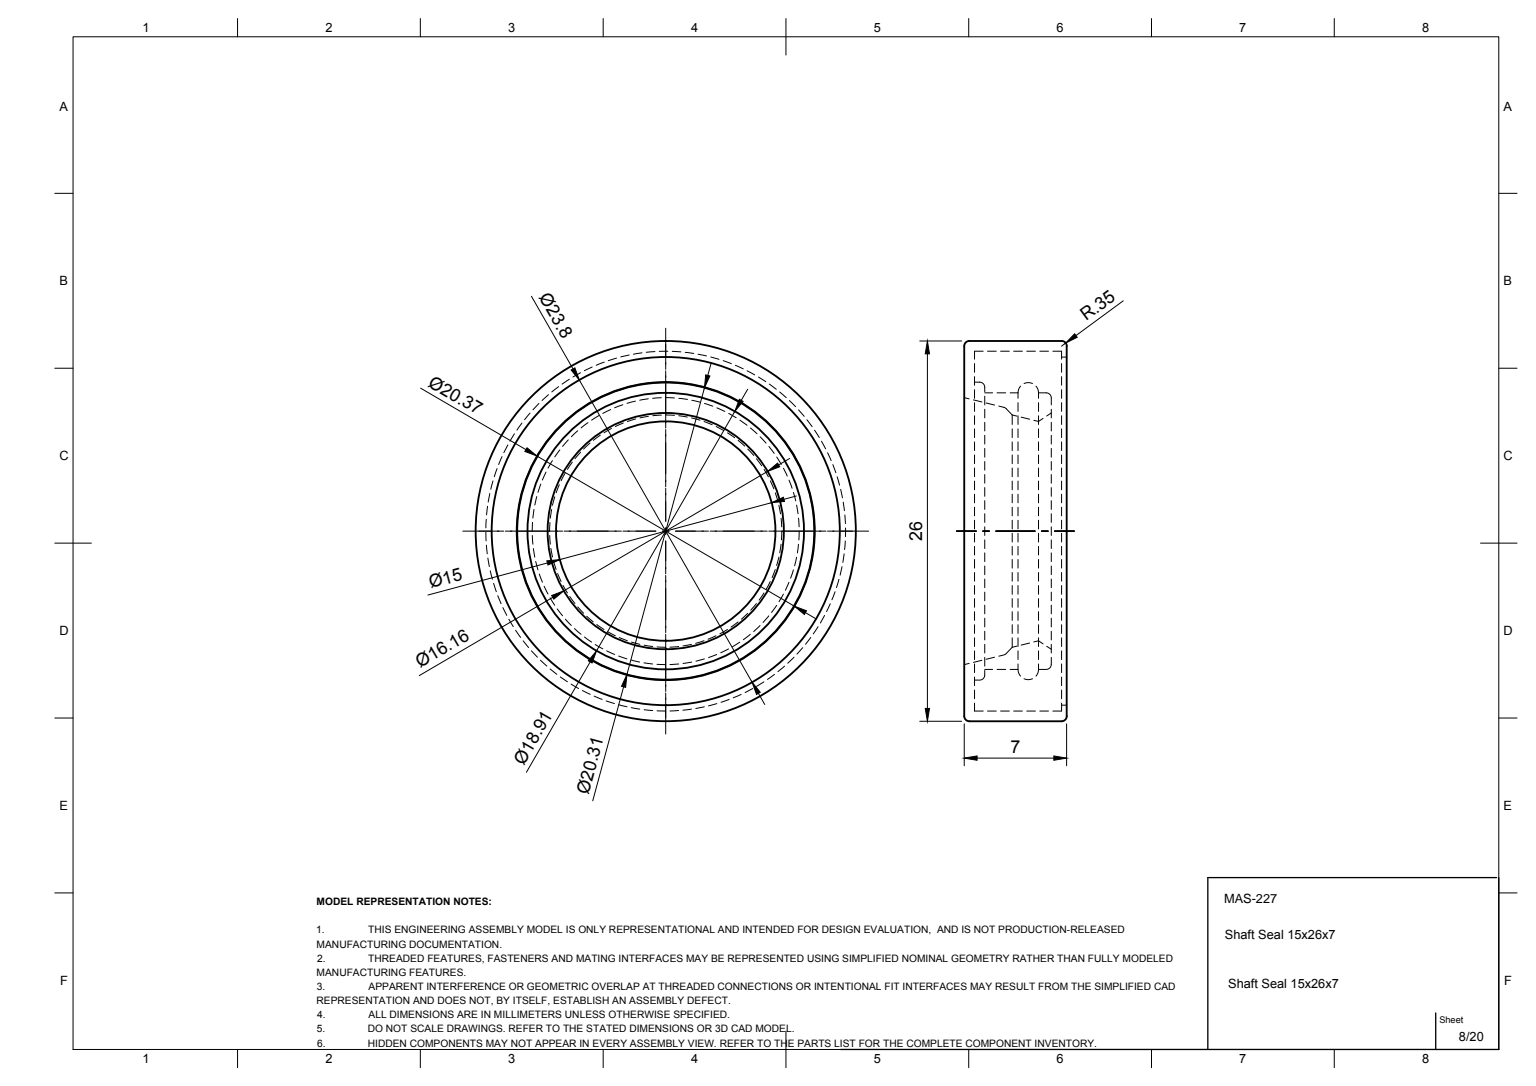
ISO-10303-21;
HEADER;
FILE_DESCRIPTION (('STEP AP214'),
    '1' );
FILE_NAME ( 'Shaft Seal 15x26x7.step', '2026-10-06T08:24:41', ( '' ), ( '' ), 'STEP AP214', 'Unspecified', '' );
FILE_SCHEMA (( 'AUTOMOTIVE_DESIGN' ));
ENDSEC;
DATA;
#41=DIRECTION ( 'NONE',  ( 0.000000000000000000, 0.000000000000000000, -1.000000000000000000 ) ) ;
#65=CARTESIAN_POINT ( 'NONE',  ( 0.000000000000000000, 0.000000000000000000, -0.2618110236220472231 ) ) ;
#81=EDGE_CURVE ( 'NONE', #10766, #14002, #19559, .T. ) ;
#117=DIRECTION ( 'NONE',  ( -1.000000000000000000, 0.000000000000000000, 0.000000000000000000 ) ) ;
#194=CARTESIAN_POINT ( 'NONE',  ( 0.000000000000000000, 0.000000000000000000, -0.2204724409448818867 ) ) ;
#212=AXIS2_PLACEMENT_3D ( 'NONE', #21327, #27824, #8463 ) ;
#213=ORIENTED_EDGE ( 'NONE', *, *, #16639, .F. ) ;
#238=SURFACE_STYLE_USAGE ( .BOTH. , #19827 ) ;
#254=CARTESIAN_POINT ( 'NONE',  ( 0.3722026523000413478, 4.558167867734008572E-17, -0.07578740157480315376 ) ) ;
#265=CIRCLE ( 'NONE', #4300, 0.01377952755905510404 ) ;
#273=AXIS2_PLACEMENT_3D ( 'NONE', #1316, #18082, #27170 ) ;
#296=EDGE_CURVE ( 'NONE', #10766, #14592, #15963, .T. ) ;
#303=DIRECTION ( 'NONE',  ( 0.000000000000000000, 0.000000000000000000, -1.000000000000000000 ) ) ;
#331=CARTESIAN_POINT ( 'NONE',  ( 0.000000000000000000, 0.000000000000000000, -0.2342519685039370358 ) ) ;
#348=EDGE_CURVE ( 'NONE', #27369, #9997, #27259, .T. ) ;
#359=DIRECTION ( 'NONE',  ( -1.000000000000000000, -1.224646799147356165E-16, 0.000000000000000000 ) ) ;
#376=CYLINDRICAL_SURFACE ( 'NONE', #17012, 0.4842519685039370358 ) ;
#434=DIRECTION ( 'NONE',  ( -1.000000000000000000, 0.000000000000000000, 0.000000000000000000 ) ) ;
#439=EDGE_LOOP ( 'NONE', ( #13382, #10561, #4608, #2891 ) ) ;
#443=CARTESIAN_POINT ( 'NONE',  ( 0.3066721922917531873, -3.755651186775971117E-17, -0.05856299212598425896 ) ) ;
#487=PRESENTATION_STYLE_ASSIGNMENT (( #238 ) ) ;
#499=DIRECTION ( 'NONE',  ( 0.000000000000000000, 0.000000000000000000, -1.000000000000000000 ) ) ;
#520=EDGE_LOOP ( 'NONE', ( #11696, #24909 ) ) ;
#533=ORIENTED_EDGE ( 'NONE', *, *, #26084, .F. ) ;
#592=ORIENTED_EDGE ( 'NONE', *, *, #21913, .F. ) ;
#630=TOROIDAL_SURFACE ( 'NONE', #15950, 0.3198827364362346048, 0.01377952755905511792 ) ;
#645=AXIS2_PLACEMENT_3D ( 'NONE', #18436, #14238, #22419 ) ;
#669=PRODUCT_DEFINITION ( 'UNKNOWN', '', #23773, #14490 ) ;
#675=EDGE_CURVE ( 'NONE', #10287, #12118, #11029, .T. ) ;
#684=AXIS2_PLACEMENT_3D ( 'NONE', #21009, #24675, #18877 ) ;
#749=DIRECTION ( 'NONE',  ( 0.000000000000000000, 0.000000000000000000, -1.000000000000000000 ) ) ;
#751=EDGE_CURVE ( 'NONE', #9997, #27369, #23688, .T. ) ;
#795=EDGE_LOOP ( 'NONE', ( #9740, #5198 ) ) ;
#821=DIRECTION ( 'NONE',  ( 0.000000000000000000, 0.000000000000000000, -1.000000000000000000 ) ) ;
#831=TOROIDAL_SURFACE ( 'NONE', #22041, 0.3584231247409862542, 0.01377952755905511792 ) ;
#855=AXIS2_PLACEMENT_3D ( 'NONE', #18013, #5044, #5477 ) ;
#862=EDGE_CURVE ( 'NONE', #24185, #27369, #15261, .T. ) ;
#879=ORIENTED_EDGE ( 'NONE', *, *, #17592, .T. ) ;
#923=ORIENTED_EDGE ( 'NONE', *, *, #17887, .T. ) ;
#963=LINE ( 'NONE', #9553, #16645 ) ;
#993=AXIS2_PLACEMENT_3D ( 'NONE', #65, #8764, #25589 ) ;
#1001=EDGE_CURVE ( 'NONE', #12118, #10287, #27735, .T. ) ;
#1023=ORIENTED_EDGE ( 'NONE', *, *, #2966, .T. ) ;
#1035=ORIENTED_EDGE ( 'NONE', *, *, #1061, .T. ) ;
#1038=AXIS2_PLACEMENT_3D ( 'NONE', #13010, #9304, #25877 ) ;
#1061=EDGE_CURVE ( 'NONE', #11368, #24827, #15560, .T. ) ;
#1071=EDGE_CURVE ( 'NONE', #14592, #10766, #7407, .T. ) ;
#1096=EDGE_CURVE ( 'NONE', #24517, #18812, #4630, .T. ) ;
#1103=CARTESIAN_POINT ( 'NONE',  ( -0.3066721922917531873, 0.000000000000000000, -0.05856299212598425896 ) ) ;
#1164=FACE_OUTER_BOUND ( 'NONE', #3351, .T. ) ;
#1242=EDGE_LOOP ( 'NONE', ( #16794, #2990 ) ) ;
#1270=FACE_OUTER_BOUND ( 'NONE', #4883, .T. ) ;
#1292=CIRCLE ( 'NONE', #4886, 0.5118110236220472231 ) ;
#1316=CARTESIAN_POINT ( 'NONE',  ( 0.000000000000000000, 0.000000000000000000, -0.05511811023622047168 ) ) ;
#1322=CARTESIAN_POINT ( 'NONE',  ( -0.3451357231661831282, 0.000000000000000000, -0.04133858267716535029 ) ) ;
#1325=VERTEX_POINT ( 'NONE', #15223 ) ;
#1343=EDGE_CURVE ( 'NONE', #22371, #24517, #19627, .T. ) ;
#1436=DIRECTION ( 'NONE',  ( 0.000000000000000000, 0.000000000000000000, -1.000000000000000000 ) ) ;
#1440=DIRECTION ( 'NONE',  ( 0.000000000000000000, 0.000000000000000000, -1.000000000000000000 ) ) ;
#1451=DIRECTION ( 'NONE',  ( -1.000000000000000000, 0.000000000000000000, 0.000000000000000000 ) ) ;
#1459=DIRECTION ( 'NONE',  ( -1.000000000000000000, 0.000000000000000000, 0.000000000000000000 ) ) ;
#1475=EDGE_LOOP ( 'NONE', ( #26767, #10716, #19172, #19322 ) ) ;
#1521=ORIENTED_EDGE ( 'NONE', *, *, #22805, .F. ) ;
#1534=EDGE_LOOP ( 'NONE', ( #26895, #14116, #21082, #6619 ) ) ;
#1556=CIRCLE ( 'NONE', #7876, 0.01377952755905510404 ) ;
#1607=CARTESIAN_POINT ( 'NONE',  ( 0.3294268239828485600, 4.034315055438739563E-17, -0.1625845656552793450 ) ) ;
#1612=ORIENTED_EDGE ( 'NONE', *, *, #7598, .F. ) ;
#1664=ORIENTED_EDGE ( 'NONE', *, *, #21562, .F. ) ;
#1690=DIRECTION ( 'NONE',  ( 0.000000000000000000, 0.000000000000000000, -1.000000000000000000 ) ) ;
#1736=DIRECTION ( 'NONE',  ( 0.000000000000000000, 0.000000000000000000, -1.000000000000000000 ) ) ;
#1759=FACE_OUTER_BOUND ( 'NONE', #17673, .T. ) ;
#1765=DIRECTION ( 'NONE',  ( 0.000000000000000000, 0.000000000000000000, -1.000000000000000000 ) ) ;
#1780=CARTESIAN_POINT ( 'NONE',  ( -0.4842519685039370358, 0.000000000000000000, -0.2480314960629921295 ) ) ;
#1842=LINE ( 'NONE', #25717, #22886 ) ;
#1850=EDGE_CURVE ( 'NONE', #14002, #24185, #9702, .T. ) ;
#1887=ORIENTED_EDGE ( 'NONE', *, *, #14871, .F. ) ;
#1940=EDGE_LOOP ( 'NONE', ( #3671, #24447, #23194, #8528 ) ) ;
#1952=VERTEX_POINT ( 'NONE', #2654 ) ;
#1999=VECTOR ( 'NONE', #24433, 39.37007874015748854 ) ;
#2097=ORIENTED_EDGE ( 'NONE', *, *, #16708, .F. ) ;
#2112=CARTESIAN_POINT ( 'NONE',  ( -0.3872945158171015589, 0.000000000000000000, -0.2204724409448818867 ) ) ;
#2132=CARTESIAN_POINT ( 'NONE',  ( -0.3722026523000413478, 0.000000000000000000, -0.1033464566929133965 ) ) ;
#2163=CARTESIAN_POINT ( 'NONE',  ( -0.5118110236220472231, 0.000000000000000000, -0.2618110236220472231 ) ) ;
#2169=ORIENTED_EDGE ( 'NONE', *, *, #348, .F. ) ;
#2180=AXIS2_PLACEMENT_3D ( 'NONE', #21071, #20654, #10050 ) ;
#2191=CARTESIAN_POINT ( 'NONE',  ( 0.000000000000000000, 0.000000000000000000, -0.2618110236220472231 ) ) ;
#2199=AXIS2_PLACEMENT_3D ( 'NONE', #24532, #20307, #18304 ) ;
#2320=FACE_OUTER_BOUND ( 'NONE', #11386, .T. ) ;
#2334=DIRECTION ( 'NONE',  ( -0.000000000000000000, -1.000000000000000000, -0.000000000000000000 ) ) ;
#2335=ORIENTED_EDGE ( 'NONE', *, *, #25585, .F. ) ;
#2415=ADVANCED_FACE ( 'NONE', ( #26187 ), #7944, .T. ) ;
#2529=ORIENTED_EDGE ( 'NONE', *, *, #26084, .T. ) ;
#2537=FACE_OUTER_BOUND ( 'NONE', #20320, .T. ) ;
#2594=DIRECTION ( 'NONE',  ( 0.000000000000000000, 0.000000000000000000, -1.000000000000000000 ) ) ;
#2606=ORIENTED_EDGE ( 'NONE', *, *, #23570, .F. ) ;
#2654=CARTESIAN_POINT ( 'NONE',  ( 0.4842519685039370358, 5.930376232091513698E-17, -0.2480314960629921295 ) ) ;
#2670=CIRCLE ( 'NONE', #22528, 0.4980314960629921295 ) ;
#2764=AXIS2_PLACEMENT_3D ( 'NONE', #194, #11024, #26267 ) ;
#2766=CARTESIAN_POINT ( 'NONE',  ( 0.000000000000000000, 0.000000000000000000, -0.01377952755905511792 ) ) ;
#2803=DIRECTION ( 'NONE',  ( -1.000000000000000000, 0.000000000000000000, 0.000000000000000000 ) ) ;
#2811=AXIS2_PLACEMENT_3D ( 'NONE', #14470, #19390, #16714 ) ;
#2837=AXIS2_PLACEMENT_3D ( 'NONE', #4234, #8058, #16514 ) ;
#2841=CARTESIAN_POINT ( 'NONE',  ( -0.3584231247409862542, 0.000000000000000000, -0.05511811023622047168 ) ) ;
#2868=DIRECTION ( 'NONE',  ( 0.000000000000000000, 0.000000000000000000, -1.000000000000000000 ) ) ;
#2891=ORIENTED_EDGE ( 'NONE', *, *, #7871, .F. ) ;
#2901=AXIS2_PLACEMENT_3D ( 'NONE', #27696, #24860, #14143 ) ;
#2907=DIRECTION ( 'NONE',  ( 0.000000000000000000, 0.000000000000000000, -1.000000000000000000 ) ) ;
#2925=( NAMED_UNIT ( * ) PLANE_ANGLE_UNIT ( ) SI_UNIT ( $, .RADIAN. ) ) ;
#2931=ORIENTED_EDGE ( 'NONE', *, *, #15459, .F. ) ;
#2966=EDGE_CURVE ( 'NONE', #10287, #1952, #26468, .T. ) ;
#2990=ORIENTED_EDGE ( 'NONE', *, *, #13862, .F. ) ;
#3078=DIRECTION ( 'NONE',  ( -1.000000000000000000, 0.000000000000000000, 0.000000000000000000 ) ) ;
#3085=UNCERTAINTY_MEASURE_WITH_UNIT (LENGTH_MEASURE( 1.000000000000000082E-05 ), #4516, 'distance_accuracy_value', 'NONE') ;
#3099=AXIS2_PLACEMENT_3D ( 'NONE', #25907, #6556, #5249 ) ;
#3113=DIRECTION ( 'NONE',  ( -1.000000000000000000, 0.000000000000000000, 0.000000000000000000 ) ) ;
#3117=VERTEX_POINT ( 'NONE', #26939 ) ;
#3156=CARTESIAN_POINT ( 'NONE',  ( 0.3722026523000413478, 4.558167867734008572E-17, -0.1756889763779527769 ) ) ;
#3246=LINE ( 'NONE', #11888, #10154 ) ;
#3260=EDGE_CURVE ( 'NONE', #24896, #24517, #12074, .T. ) ;
#3264=ORIENTED_EDGE ( 'NONE', *, *, #19902, .T. ) ;
#3351=EDGE_LOOP ( 'NONE', ( #1612, #533, #23574, #1035 ) ) ;
#3364=CIRCLE ( 'NONE', #24588, 0.4685039370078740717 ) ;
#3375=DIRECTION ( 'NONE',  ( -1.224646799147353207E-16, 1.000000000000000000, 0.000000000000000000 ) ) ;
#3414=CARTESIAN_POINT ( 'NONE',  ( 0.4010740433761567081, 4.911740434416970370E-17, -0.2480314960629921295 ) ) ;
#3449=PRODUCT ( 'Shaft Seal 15x26x7', 'Shaft Seal 15x26x7', '', ( #15092 ) ) ;
#3500=EDGE_CURVE ( 'NONE', #23791, #1325, #26299, .T. ) ;
#3545=CONICAL_SURFACE ( 'NONE', #3099, 0.3224687058348476576, 0.8056700744428512140 ) ;
#3574=ADVANCED_FACE ( 'NONE', ( #8255 ), #831, .T. ) ;
#3605=LINE ( 'NONE', #16340, #11324 ) ;
#3619=DIRECTION ( 'NONE',  ( 0.000000000000000000, 0.000000000000000000, -1.000000000000000000 ) ) ;
#3632=CARTESIAN_POINT ( 'NONE',  ( 0.000000000000000000, 0.000000000000000000, -0.2480314960629921295 ) ) ;
#3665=DIRECTION ( 'NONE',  ( 0.000000000000000000, 0.000000000000000000, 1.000000000000000000 ) ) ;
#3671=ORIENTED_EDGE ( 'NONE', *, *, #6583, .T. ) ;
#3747=AXIS2_PLACEMENT_3D ( 'NONE', #13845, #13696, #27128 ) ;
#3757=DIRECTION ( 'NONE',  ( 1.000000000000000000, 0.000000000000000000, 0.000000000000000000 ) ) ;
#3774=CARTESIAN_POINT ( 'NONE',  ( 0.000000000000000000, 0.000000000000000000, -0.2342519685039370358 ) ) ;
#3782=VERTEX_POINT ( 'NONE', #27226 ) ;
#3860=ORIENTED_EDGE ( 'NONE', *, *, #12938, .F. ) ;
#3869=AXIS2_PLACEMENT_3D ( 'NONE', #13603, #22220, #24208 ) ;
#3928=DIRECTION ( 'NONE',  ( -1.000000000000000000, 0.000000000000000000, 0.000000000000000000 ) ) ;
#3959=FACE_BOUND ( 'NONE', #21442, .T. ) ;
#3969=ADVANCED_FACE ( 'NONE', ( #25527 ), #18427, .T. ) ;
#3988=AXIS2_PLACEMENT_3D ( 'NONE', #5088, #13709, #17926 ) ;
#4011=VECTOR ( 'NONE', #2594, 39.37007874015748143 ) ;
#4034=ORIENTED_EDGE ( 'NONE', *, *, #13927, .F. ) ;
#4073=EDGE_LOOP ( 'NONE', ( #12359, #15976, #13179, #213 ) ) ;
#4076=ORIENTED_EDGE ( 'NONE', *, *, #6993, .T. ) ;
#4085=DIRECTION ( 'NONE',  ( 0.000000000000000000, 0.000000000000000000, -1.000000000000000000 ) ) ;
#4131=ORIENTED_EDGE ( 'NONE', *, *, #8880, .F. ) ;
#4152=EDGE_CURVE ( 'NONE', #18288, #1952, #14403, .T. ) ;
#4159=EDGE_CURVE ( 'NONE', #12825, #16461, #23873, .T. ) ;
#4174=DIRECTION ( 'NONE',  ( -1.000000000000000000, 0.000000000000000000, 0.000000000000000000 ) ) ;
#4185=EDGE_CURVE ( 'NONE', #24622, #11368, #963, .T. ) ;
#4198=DIRECTION ( 'NONE',  ( 1.000000000000000000, 0.000000000000000000, 0.000000000000000000 ) ) ;
#4205=VERTEX_POINT ( 'NONE', #11407 ) ;
#4234=CARTESIAN_POINT ( 'NONE',  ( 0.000000000000000000, 0.000000000000000000, -0.04133858267716535029 ) ) ;
#4243=ORIENTED_EDGE ( 'NONE', *, *, #3500, .T. ) ;
#4258=EDGE_CURVE ( 'NONE', #24011, #9956, #2670, .T. ) ;
#4300=AXIS2_PLACEMENT_3D ( 'NONE', #16529, #3375, #25007 ) ;
#4306=LENGTH_MEASURE_WITH_UNIT ( LENGTH_MEASURE( 0.02539999999999999897 ), #16546 ) ;
#4362=FACE_BOUND ( 'NONE', #16942, .T. ) ;
#4391=TOROIDAL_SURFACE ( 'NONE', #13855, 0.4980314960629921295, 0.01377952755905511792 ) ;
#4495=ORIENTED_EDGE ( 'NONE', *, *, #4565, .F. ) ;
#4514=ORIENTED_EDGE ( 'NONE', *, *, #12938, .T. ) ;
#4516=( CONVERSION_BASED_UNIT ( 'INCH', #17637 ) LENGTH_UNIT ( ) NAMED_UNIT ( #13045 ) ) ;
#4522=AXIS2_PLACEMENT_3D ( 'NONE', #23164, #4085, #12689 ) ;
#4543=FACE_OUTER_BOUND ( 'NONE', #439, .T. ) ;
#4565=EDGE_CURVE ( 'NONE', #19035, #26909, #23390, .T. ) ;
#4608=ORIENTED_EDGE ( 'NONE', *, *, #25493, .T. ) ;
#4630=LINE ( 'NONE', #11409, #27280 ) ;
#4651=CARTESIAN_POINT ( 'NONE',  ( -0.4980314960629921295, 0.000000000000000000, -0.01377952755905511792 ) ) ;
#4653=AXIS2_PLACEMENT_3D ( 'NONE', #8465, #16949, #17084 ) ;
#4658=DIRECTION ( 'NONE',  ( 0.000000000000000000, 0.000000000000000000, -1.000000000000000000 ) ) ;
#4672=ORIENTED_EDGE ( 'NONE', *, *, #20993, .F. ) ;
#4698=VECTOR ( 'NONE', #25982, 39.37007874015748143 ) ;
#4709=FACE_OUTER_BOUND ( 'NONE', #18885, .T. ) ;
#4717=CARTESIAN_POINT ( 'NONE',  ( 0.4980314960629921295, 6.099126775281109802E-17, -0.2618110236220472231 ) ) ;
#4744=EDGE_CURVE ( 'NONE', #23791, #26519, #25173, .T. ) ;
#4758=DIRECTION ( 'NONE',  ( -1.000000000000000000, 0.000000000000000000, 0.000000000000000000 ) ) ;
#4790=CARTESIAN_POINT ( 'NONE',  ( -0.3872945158171015589, 0.000000000000000000, -0.2342519685039370358 ) ) ;
#4797=DIRECTION ( 'NONE',  ( 0.000000000000000000, 0.000000000000000000, -1.000000000000000000 ) ) ;
#4813=CYLINDRICAL_SURFACE ( 'NONE', #23754, 0.4842519685039370358 ) ;
#4818=PLANE ( 'NONE',  #10795 ) ;
#4883=EDGE_LOOP ( 'NONE', ( #25142, #5686, #879, #22401 ) ) ;
#4886=AXIS2_PLACEMENT_3D ( 'NONE', #20717, #18864, #3757 ) ;
#4900=CIRCLE ( 'NONE', #8520, 0.01377952755905510404 ) ;
#4917=ORIENTED_EDGE ( 'NONE', *, *, #24991, .T. ) ;
#4922=DIRECTION ( 'NONE',  ( 0.000000000000000000, 0.000000000000000000, -1.000000000000000000 ) ) ;
#4938=LINE ( 'NONE', #16481, #5532 ) ;
#4960=ORIENTED_EDGE ( 'NONE', *, *, #17477, .T. ) ;
#4971=DIRECTION ( 'NONE',  ( -1.224646799147353207E-16, 1.000000000000000000, 0.000000000000000000 ) ) ;
#4989=DIRECTION ( 'NONE',  ( -1.000000000000000000, -1.224646799147356165E-16, 0.000000000000000000 ) ) ;
#5022=ORIENTED_EDGE ( 'NONE', *, *, #1850, .F. ) ;
#5038=FACE_OUTER_BOUND ( 'NONE', #20604, .T. ) ;
#5044=DIRECTION ( 'NONE',  ( 0.000000000000000000, 0.000000000000000000, -1.000000000000000000 ) ) ;
#5065=PLANE ( 'NONE',  #10827 ) ;
#5088=CARTESIAN_POINT ( 'NONE',  ( 0.000000000000000000, 0.000000000000000000, -0.2480314960629921295 ) ) ;
#5132=CARTESIAN_POINT ( 'NONE',  ( 0.000000000000000000, 0.000000000000000000, -0.2480314960629921295 ) ) ;
#5142=EDGE_CURVE ( 'NONE', #26728, #9665, #11645, .T. ) ;
#5157=CARTESIAN_POINT ( 'NONE',  ( -0.3180687940157840843, 0.000000000000000000, -0.04133858267716535029 ) ) ;
#5172=DIRECTION ( 'NONE',  ( 0.000000000000000000, 0.000000000000000000, -1.000000000000000000 ) ) ;
#5198=ORIENTED_EDGE ( 'NONE', *, *, #4258, .F. ) ;
#5209=FACE_BOUND ( 'NONE', #24077, .T. ) ;
#5229=CARTESIAN_POINT ( 'NONE',  ( 0.000000000000000000, 0.000000000000000000, 0.000000000000000000 ) ) ;
#5249=DIRECTION ( 'NONE',  ( -1.000000000000000000, 0.000000000000000000, 0.000000000000000000 ) ) ;
#5324=DIRECTION ( 'NONE',  ( 0.000000000000000000, 0.000000000000000000, -1.000000000000000000 ) ) ;
#5362=EDGE_CURVE ( 'NONE', #24896, #5769, #7155, .T. ) ;
#5426=DIRECTION ( 'NONE',  ( 0.000000000000000000, 0.000000000000000000, -1.000000000000000000 ) ) ;
#5435=DIRECTION ( 'NONE',  ( -1.224646799147353207E-16, 1.000000000000000000, 0.000000000000000000 ) ) ;
#5475=ORIENTED_EDGE ( 'NONE', *, *, #19235, .T. ) ;
#5477=DIRECTION ( 'NONE',  ( -1.000000000000000000, 0.000000000000000000, 0.000000000000000000 ) ) ;
#5526=CARTESIAN_POINT ( 'NONE',  ( -0.3294268239828485600, 0.000000000000000000, -0.1625845656552793450 ) ) ;
#5532=VECTOR ( 'NONE', #13554, 39.37007874015748143 ) ;
#5536=CARTESIAN_POINT ( 'NONE',  ( -0.4980314960629921295, 0.000000000000000000, -6.010066929133858501E-17 ) ) ;
#5627=AXIS2_PLACEMENT_3D ( 'NONE', #7311, #11547, #26653 ) ;
#5653=DIRECTION ( 'NONE',  ( 0.000000000000000000, 0.000000000000000000, 1.000000000000000000 ) ) ;
#5668=CYLINDRICAL_SURFACE ( 'NONE', #16513, 0.5118110236220472231 ) ;
#5686=ORIENTED_EDGE ( 'NONE', *, *, #348, .T. ) ;
#5769=VERTEX_POINT ( 'NONE', #2112 ) ;
#5792=DIRECTION ( 'NONE',  ( 0.2384530002628495460, 2.920207035189816837E-17, -0.9711540385879292581 ) ) ;
#5808=ORIENTED_EDGE ( 'NONE', *, *, #17183, .T. ) ;
#5833=CARTESIAN_POINT ( 'NONE',  ( 0.000000000000000000, 0.000000000000000000, -0.1309055118110236116 ) ) ;
#5841=AXIS2_PLACEMENT_3D ( 'NONE', #9381, #11656, #26442 ) ;
#5879=AXIS2_PLACEMENT_3D ( 'NONE', #10428, #19043, #27677 ) ;
#5923=ORIENTED_EDGE ( 'NONE', *, *, #14871, .T. ) ;
#5944=CARTESIAN_POINT ( 'NONE',  ( 0.000000000000000000, 0.000000000000000000, -0.07578740157480315376 ) ) ;
#5950=EDGE_CURVE ( 'NONE', #7273, #4205, #13910, .T. ) ;
#5972=CYLINDRICAL_SURFACE ( 'NONE', #15485, 0.3722026523000413478 ) ;
#5974=CARTESIAN_POINT ( 'NONE',  ( 0.000000000000000000, 0.000000000000000000, -0.07578740157480315376 ) ) ;
#5976=PRODUCT_DEFINITION_SHAPE ( 'NONE', 'NONE',  #669 ) ;
#6046=EDGE_CURVE ( 'NONE', #24011, #26909, #17569, .T. ) ;
#6071=ORIENTED_EDGE ( 'NONE', *, *, #1061, .F. ) ;
#6081=ADVANCED_FACE ( 'NONE', ( #8664 ), #3545, .F. ) ;
#6095=AXIS2_PLACEMENT_3D ( 'NONE', #19887, #2907, #17877 ) ;
#6167=DIRECTION ( 'NONE',  ( 0.000000000000000000, 0.000000000000000000, -1.000000000000000000 ) ) ;
#6215=( GEOMETRIC_REPRESENTATION_CONTEXT ( 3 ) GLOBAL_UNCERTAINTY_ASSIGNED_CONTEXT ( ( #3085 ) ) GLOBAL_UNIT_ASSIGNED_CONTEXT ( ( #4516, #2925, #13530 ) ) REPRESENTATION_CONTEXT ( 'NONE', 'WORKASPACE' ) ) ;
#6217=DIRECTION ( 'NONE',  ( 0.000000000000000000, 0.000000000000000000, -1.000000000000000000 ) ) ;
#6258=ORIENTED_EDGE ( 'NONE', *, *, #6939, .T. ) ;
#6298=ADVANCED_FACE ( 'NONE', ( #24808 ), #21203, .F. ) ;
#6346=CIRCLE ( 'NONE', #22111, 0.3126261861498082495 ) ;
#6408=VECTOR ( 'NONE', #23622, 39.37007874015748143 ) ;
#6511=CARTESIAN_POINT ( 'NONE',  ( 0.000000000000000000, 0.000000000000000000, -0.2755905511811023723 ) ) ;
#6516=DIRECTION ( 'NONE',  ( 0.000000000000000000, 0.000000000000000000, -1.000000000000000000 ) ) ;
#6522=DIRECTION ( 'NONE',  ( -1.000000000000000000, 0.000000000000000000, 0.000000000000000000 ) ) ;
#6549=ADVANCED_FACE ( 'NONE', ( #22241 ), #11271, .F. ) ;
#6556=DIRECTION ( 'NONE',  ( 0.000000000000000000, 0.000000000000000000, -1.000000000000000000 ) ) ;
#6583=EDGE_CURVE ( 'NONE', #25216, #7273, #13982, .T. ) ;
#6619=ORIENTED_EDGE ( 'NONE', *, *, #1343, .T. ) ;
#6642=SHAPE_REPRESENTATION_RELATIONSHIP ( 'NONE' , 'NONE' ,  #25798, #26182 ) ;
#6643=EDGE_LOOP ( 'NONE', ( #22688, #22613, #16731, #9252 ) ) ;
#6647=ORIENTED_EDGE ( 'NONE', *, *, #4744, .F. ) ;
#6698=AXIS2_PLACEMENT_3D ( 'NONE', #2766, #5172, #4758 ) ;
#6772=CARTESIAN_POINT ( 'NONE',  ( 0.000000000000000000, 0.000000000000000000, -0.04133858267716535029 ) ) ;
#6782=CIRCLE ( 'NONE', #5879, 0.4980314960629921295 ) ;
#6810=ORIENTED_EDGE ( 'NONE', *, *, #24229, .T. ) ;
#6817=DIRECTION ( 'NONE',  ( 1.000000000000000000, 0.000000000000000000, 0.000000000000000000 ) ) ;
#6838=ADVANCED_FACE ( 'NONE', ( #5209, #24420 ), #5065, .T. ) ;
#6882=CARTESIAN_POINT ( 'NONE',  ( 0.000000000000000000, 0.000000000000000000, -0.04133858267716535029 ) ) ;
#6908=AXIS2_PLACEMENT_3D ( 'NONE', #331, #22179, #2803 ) ;
#6939=EDGE_CURVE ( 'NONE', #13078, #3782, #9931, .T. ) ;
#6944=CARTESIAN_POINT ( 'NONE',  ( 0.000000000000000000, 0.000000000000000000, -0.05511811023622047168 ) ) ;
#6955=DIRECTION ( 'NONE',  ( 0.000000000000000000, 0.000000000000000000, 1.000000000000000000 ) ) ;
#6961=FACE_BOUND ( 'NONE', #20194, .T. ) ;
#6993=EDGE_CURVE ( 'NONE', #24685, #19453, #6782, .T. ) ;
#7035=DIRECTION ( 'NONE',  ( -0.5518027697606309179, 0.000000000000000000, 0.8339746418713797071 ) ) ;
#7075=CARTESIAN_POINT ( 'NONE',  ( 0.4980314960629921295, 6.183502046875907854E-17, -6.010066929133858501E-17 ) ) ;
#7155=CIRCLE ( 'NONE', #20236, 0.3872945158171015589 ) ;
#7209=CIRCLE ( 'NONE', #9453, 0.4685039370078740717 ) ;
#7216=ORIENTED_EDGE ( 'NONE', *, *, #19235, .F. ) ;
#7240=DIRECTION ( 'NONE',  ( 0.000000000000000000, 0.000000000000000000, -1.000000000000000000 ) ) ;
#7251=DIRECTION ( 'NONE',  ( -1.224646799147353207E-16, 1.000000000000000000, 0.000000000000000000 ) ) ;
#7269=CIRCLE ( 'NONE', #23083, 0.3126261861498082495 ) ;
#7273=VERTEX_POINT ( 'NONE', #10850 ) ;
#7294=ORIENTED_EDGE ( 'NONE', *, *, #18218, .F. ) ;
#7311=CARTESIAN_POINT ( 'NONE',  ( 0.000000000000000000, 0.000000000000000000, -0.01377952755905511792 ) ) ;
#7319=FACE_OUTER_BOUND ( 'NONE', #20969, .T. ) ;
#7335=DIRECTION ( 'NONE',  ( 0.000000000000000000, 0.000000000000000000, -1.000000000000000000 ) ) ;
#7337=LINE ( 'NONE', #20334, #12740 ) ;
#7340=CONICAL_SURFACE ( 'NONE', #1038, 0.3458446900868161200, 0.2407725888118960322 ) ;
#7389=ORIENTED_EDGE ( 'NONE', *, *, #17516, .F. ) ;
#7401=DIRECTION ( 'NONE',  ( 0.000000000000000000, 0.000000000000000000, -1.000000000000000000 ) ) ;
#7407=CIRCLE ( 'NONE', #21421, 0.3584231247409862542 ) ;
#7429=ORIENTED_EDGE ( 'NONE', *, *, #14472, .F. ) ;
#7435=AXIS2_PLACEMENT_3D ( 'NONE', #21554, #26202, #17317 ) ;
#7573=ORIENTED_EDGE ( 'NONE', *, *, #4152, .F. ) ;
#7598=EDGE_CURVE ( 'NONE', #20206, #24827, #3605, .T. ) ;
#7620=ORIENTED_EDGE ( 'NONE', *, *, #296, .F. ) ;
#7772=DIRECTION ( 'NONE',  ( 0.000000000000000000, 0.000000000000000000, 1.000000000000000000 ) ) ;
#7828=CONICAL_SURFACE ( 'NONE', #17300, 0.3039508883504944969, 0.2407725888118948110 ) ;
#7871=EDGE_CURVE ( 'NONE', #18812, #10946, #13575, .T. ) ;
#7876=AXIS2_PLACEMENT_3D ( 'NONE', #8330, #25560, #6217 ) ;
#7895=ORIENTED_EDGE ( 'NONE', *, *, #17101, .T. ) ;
#7923=DIRECTION ( 'NONE',  ( 1.000000000000000000, 0.000000000000000000, 0.000000000000000000 ) ) ;
#7928=FACE_OUTER_BOUND ( 'NONE', #14771, .T. ) ;
#7929=CARTESIAN_POINT ( 'NONE',  ( 0.4842519685039370358, 5.930376232091513698E-17, -0.01377952755905511792 ) ) ;
#7939=ORIENTED_EDGE ( 'NONE', *, *, #1071, .F. ) ;
#7944=TOROIDAL_SURFACE ( 'NONE', #3869, 0.3872945158171015589, 0.01377952755905511792 ) ;
#8035=ORIENTED_EDGE ( 'NONE', *, *, #751, .F. ) ;
#8053=CARTESIAN_POINT ( 'NONE',  ( 0.4685039370078740717, 5.737518468446261360E-17, -0.01377952755905511792 ) ) ;
#8058=DIRECTION ( 'NONE',  ( 0.000000000000000000, 0.000000000000000000, -1.000000000000000000 ) ) ;
#8068=CIRCLE ( 'NONE', #3988, 0.4010740433761567081 ) ;
#8091=DIRECTION ( 'NONE',  ( 1.000000000000000000, 0.000000000000000000, 0.000000000000000000 ) ) ;
#8136=CARTESIAN_POINT ( 'NONE',  ( 0.000000000000000000, 0.000000000000000000, -0.1033464566929133965 ) ) ;
#8187=FACE_OUTER_BOUND ( 'NONE', #22720, .T. ) ;
#8245=ORIENTED_EDGE ( 'NONE', *, *, #675, .T. ) ;
#8255=FACE_OUTER_BOUND ( 'NONE', #17710, .T. ) ;
#8267=CARTESIAN_POINT ( 'NONE',  ( 0.000000000000000000, 0.000000000000000000, -0.2618110236220472231 ) ) ;
#8275=CIRCLE ( 'NONE', #22260, 0.3180687940323247975 ) ;
#8330=CARTESIAN_POINT ( 'NONE',  ( -0.3198827364362346048, 0.000000000000000000, -0.1725236688546921415 ) ) ;
#8341=CARTESIAN_POINT ( 'NONE',  ( 0.3722026523000413478, 4.558167867734008572E-17, -0.05856299212598425896 ) ) ;
#8355=ORIENTED_EDGE ( 'NONE', *, *, #17101, .F. ) ;
#8379=VECTOR ( 'NONE', #7240, 39.37007874015748143 ) ;
#8402=CIRCLE ( 'NONE', #19696, 0.3722026523000413478 ) ;
#8463=DIRECTION ( 'NONE',  ( -1.000000000000000000, 0.000000000000000000, 0.000000000000000000 ) ) ;
#8465=CARTESIAN_POINT ( 'NONE',  ( 0.000000000000000000, 0.000000000000000000, -0.01377952755905511792 ) ) ;
#8515=EDGE_LOOP ( 'NONE', ( #592, #18928, #22938, #7216 ) ) ;
#8520=AXIS2_PLACEMENT_3D ( 'NONE', #4717, #7251, #4989 ) ;
#8521=DIRECTION ( 'NONE',  ( 0.2384530002628483802, 2.920207035189802662E-17, -0.9711540385879295911 ) ) ;
#8528=ORIENTED_EDGE ( 'NONE', *, *, #20884, .F. ) ;
#8592=VERTEX_POINT ( 'NONE', #11189 ) ;
#8664=FACE_OUTER_BOUND ( 'NONE', #8515, .T. ) ;
#8709=SHAPE_DEFINITION_REPRESENTATION ( #5976, #25798 ) ;
#8714=AXIS2_PLACEMENT_3D ( 'NONE', #15823, #5653, #14277 ) ;
#8717=EDGE_LOOP ( 'NONE', ( #12154, #5022, #11792, #2169 ) ) ;
#8764=DIRECTION ( 'NONE',  ( 0.000000000000000000, 0.000000000000000000, -1.000000000000000000 ) ) ;
#8873=DIRECTION ( 'NONE',  ( -1.000000000000000000, 0.000000000000000000, 0.000000000000000000 ) ) ;
#8880=EDGE_CURVE ( 'NONE', #19062, #17310, #13156, .T. ) ;
#9017=ADVANCED_FACE ( 'NONE', ( #2537 ), #11381, .F. ) ;
#9042=CYLINDRICAL_SURFACE ( 'NONE', #6908, 0.4010740433761567081 ) ;
#9047=CARTESIAN_POINT ( 'NONE',  ( -0.5118110236220472231, 0.000000000000000000, -0.1377952755905511861 ) ) ;
#9080=CIRCLE ( 'NONE', #2764, 0.3872945158171015589 ) ;
#9088=ORIENTED_EDGE ( 'NONE', *, *, #25383, .T. ) ;
#9105=EDGE_CURVE ( 'NONE', #13078, #16461, #7337, .T. ) ;
#9114=ORIENTED_EDGE ( 'NONE', *, *, #2966, .F. ) ;
#9149=EDGE_LOOP ( 'NONE', ( #26444, #21592, #9088, #24473 ) ) ;
#9157=EDGE_LOOP ( 'NONE', ( #18455, #8245 ) ) ;
#9252=ORIENTED_EDGE ( 'NONE', *, *, #25493, .F. ) ;
#9289=CARTESIAN_POINT ( 'NONE',  ( 0.000000000000000000, 0.000000000000000000, -0.01377952755905511792 ) ) ;
#9304=DIRECTION ( 'NONE',  ( 0.000000000000000000, 0.000000000000000000, -1.000000000000000000 ) ) ;
#9338=DIRECTION ( 'NONE',  ( -1.000000000000000000, 0.000000000000000000, 0.000000000000000000 ) ) ;
#9379=ORIENTED_EDGE ( 'NONE', *, *, #15719, .F. ) ;
#9381=CARTESIAN_POINT ( 'NONE',  ( 0.000000000000000000, 0.000000000000000000, -0.01377952755905511792 ) ) ;
#9453=AXIS2_PLACEMENT_3D ( 'NONE', #9289, #25084, #15553 ) ;
#9543=DIRECTION ( 'NONE',  ( -1.000000000000000000, 0.000000000000000000, 0.000000000000000000 ) ) ;
#9553=CARTESIAN_POINT ( 'NONE',  ( -0.4685039370078740717, 0.000000000000000000, -0.006889763779527558960 ) ) ;
#9570=FACE_OUTER_BOUND ( 'NONE', #13886, .T. ) ;
#9603=VECTOR ( 'NONE', #7035, 39.37007874015748143 ) ;
#9614=CYLINDRICAL_SURFACE ( 'NONE', #15941, 0.4685039370078740717 ) ;
#9665=VERTEX_POINT ( 'NONE', #1607 ) ;
#9702=CIRCLE ( 'NONE', #273, 0.3722026523000413478 ) ;
#9740=ORIENTED_EDGE ( 'NONE', *, *, #13812, .F. ) ;
#9770=CARTESIAN_POINT ( 'NONE',  ( -0.4685039370078740717, 0.000000000000000000, -6.283251968503937502E-17 ) ) ;
#9795=CARTESIAN_POINT ( 'NONE',  ( 0.000000000000000000, 0.000000000000000000, -0.1377952755905511861 ) ) ;
#9870=EDGE_LOOP ( 'NONE', ( #14412, #13682, #19670, #20142 ) ) ;
#9927=VECTOR ( 'NONE', #8521, 39.37007874015748854 ) ;
#9931=CIRCLE ( 'NONE', #4522, 0.3332647802741406373 ) ;
#9956=VERTEX_POINT ( 'NONE', #5536 ) ;
#9982=AXIS2_PLACEMENT_3D ( 'NONE', #10313, #18935, #12448 ) ;
#9983=ADVANCED_FACE ( 'NONE', ( #1164 ), #9614, .F. ) ;
#9997=VERTEX_POINT ( 'NONE', #26708 ) ;
#10006=EDGE_LOOP ( 'NONE', ( #7620, #7939 ) ) ;
#10050=DIRECTION ( 'NONE',  ( 1.000000000000000000, 0.000000000000000000, 0.000000000000000000 ) ) ;
#10054=TOROIDAL_SURFACE ( 'NONE', #24485, 0.3584231247409862542, 0.01377952755905511792 ) ;
#10060=DIRECTION ( 'NONE',  ( 0.000000000000000000, 0.000000000000000000, -1.000000000000000000 ) ) ;
#10108=ORIENTED_EDGE ( 'NONE', *, *, #4159, .F. ) ;
#10154=VECTOR ( 'NONE', #20507, 39.37007874015748143 ) ;
#10177=ORIENTED_EDGE ( 'NONE', *, *, #14019, .F. ) ;
#10247=CARTESIAN_POINT ( 'NONE',  ( -0.3722026523000413478, 0.000000000000000000, -0.1309055118110236116 ) ) ;
#10259=DIRECTION ( 'NONE',  ( 1.000000000000000000, 0.000000000000000000, 0.000000000000000000 ) ) ;
#10287=VERTEX_POINT ( 'NONE', #7929 ) ;
#10313=CARTESIAN_POINT ( 'NONE',  ( 0.000000000000000000, 0.000000000000000000, -0.05856299212598425896 ) ) ;
#10323=CARTESIAN_POINT ( 'NONE',  ( -0.4010740433761567081, 0.000000000000000000, -0.2342519685039370358 ) ) ;
#10329=CARTESIAN_POINT ( 'NONE',  ( 0.000000000000000000, 0.000000000000000000, -0.1756889763779527769 ) ) ;
#10355=AXIS2_PLACEMENT_3D ( 'NONE', #4651, #13277, #14875 ) ;
#10412=EDGE_LOOP ( 'NONE', ( #19833, #923, #11295, #20248 ) ) ;
#10419=AXIS2_PLACEMENT_3D ( 'NONE', #5132, #7401, #20254 ) ;
#10428=CARTESIAN_POINT ( 'NONE',  ( 0.000000000000000000, 0.000000000000000000, -0.2755905511811023723 ) ) ;
#10450=DIRECTION ( 'NONE',  ( -0.7212949172625979788, 0.000000000000000000, -0.6926280692631088254 ) ) ;
#10476=CARTESIAN_POINT ( 'NONE',  ( -0.4842519685039370358, 0.000000000000000000, -0.01377952755905511792 ) ) ;
#10487=DIRECTION ( 'NONE',  ( -1.000000000000000000, 0.000000000000000000, 0.000000000000000000 ) ) ;
#10493=CIRCLE ( 'NONE', #2811, 0.01377952755905510404 ) ;
#10522=CIRCLE ( 'NONE', #3747, 0.4980314960629921295 ) ;
#10527=TOROIDAL_SURFACE ( 'NONE', #212, 0.3198827364362346048, 0.01377952755905511792 ) ;
#10541=CIRCLE ( 'NONE', #2837, 0.3180687940323247975 ) ;
#10546=ORIENTED_EDGE ( 'NONE', *, *, #20884, .T. ) ;
#10555=AXIS2_PLACEMENT_3D ( 'NONE', #5974, #11899, #18952 ) ;
#10561=ORIENTED_EDGE ( 'NONE', *, *, #1343, .F. ) ;
#10573=AXIS2_PLACEMENT_3D ( 'NONE', #5944, #27407, #16254 ) ;
#10579=CYLINDRICAL_SURFACE ( 'NONE', #20062, 0.4010740433761567081 ) ;
#10598=DIRECTION ( 'NONE',  ( -0.000000000000000000, -1.000000000000000000, -0.000000000000000000 ) ) ;
#10626=VERTEX_POINT ( 'NONE', #5157 ) ;
#10692=ORIENTED_EDGE ( 'NONE', *, *, #27699, .F. ) ;
#10693=CIRCLE ( 'NONE', #14311, 0.3722026523000413478 ) ;
#10716=ORIENTED_EDGE ( 'NONE', *, *, #6939, .F. ) ;
#10719=MECHANICAL_DESIGN_GEOMETRIC_PRESENTATION_REPRESENTATION('',(#22902),#12971);
#10755=CARTESIAN_POINT ( 'NONE',  ( 0.000000000000000000, 0.000000000000000000, -0.07578740157480315376 ) ) ;
#10766=VERTEX_POINT ( 'NONE', #27208 ) ;
#10790=VECTOR ( 'NONE', #26899, 39.37007874015748143 ) ;
#10795=AXIS2_PLACEMENT_3D ( 'NONE', #19396, #19679, #21521 ) ;
#10799=SURFACE_STYLE_FILL_AREA ( #23802 ) ;
#10803=CARTESIAN_POINT ( 'NONE',  ( -0.5118110236220472231, 0.000000000000000000, -0.01377952755905511792 ) ) ;
#10824=CONICAL_SURFACE ( 'NONE', #18947, 0.3066721922917531873, 0.5845243560369969282 ) ;
#10827=AXIS2_PLACEMENT_3D ( 'NONE', #22307, #7335, #15953 ) ;
#10845=ADVANCED_FACE ( 'NONE', ( #18562 ), #20862, .T. ) ;
#10850=CARTESIAN_POINT ( 'NONE',  ( 0.3722026523000413478, 4.558167867734008572E-17, -0.1309055118110236116 ) ) ;
#10920=DIRECTION ( 'NONE',  ( -0.2384530002628483802, 0.000000000000000000, -0.9711540385879295911 ) ) ;
#10946=VERTEX_POINT ( 'NONE', #13190 ) ;
#10974=ORIENTED_EDGE ( 'NONE', *, *, #22805, .T. ) ;
#11006=AXIS2_PLACEMENT_3D ( 'NONE', #20795, #1440, #8091 ) ;
#11024=DIRECTION ( 'NONE',  ( 0.000000000000000000, 0.000000000000000000, -1.000000000000000000 ) ) ;
#11029=CIRCLE ( 'NONE', #14668, 0.4842519685039370358 ) ;
#11089=DIRECTION ( 'NONE',  ( 0.000000000000000000, 0.000000000000000000, -1.000000000000000000 ) ) ;
#11167=AXIS2_PLACEMENT_3D ( 'NONE', #23487, #10598, #21060 ) ;
#11189=CARTESIAN_POINT ( 'NONE',  ( 0.3126261861395013275, 3.828566581853849315E-17, -0.1464516454673935042 ) ) ;
#11215=EDGE_CURVE ( 'NONE', #14592, #24185, #10493, .T. ) ;
#11267=CARTESIAN_POINT ( 'NONE',  ( 0.3872945158171015589, 4.827365162822171701E-17, -0.2204724409448818867 ) ) ;
#11271=CONICAL_SURFACE ( 'NONE', #14436, 0.3458446900868161200, 0.2407725888118960322 ) ;
#11295=ORIENTED_EDGE ( 'NONE', *, *, #4159, .T. ) ;
#11315=DIRECTION ( 'NONE',  ( -1.000000000000000000, 0.000000000000000000, 0.000000000000000000 ) ) ;
#11324=VECTOR ( 'NONE', #25087, 39.37007874015748143 ) ;
#11367=CARTESIAN_POINT ( 'NONE',  ( 0.000000000000000000, 0.000000000000000000, -0.2204724409448818867 ) ) ;
#11368=VERTEX_POINT ( 'NONE', #21200 ) ;
#11381=CONICAL_SURFACE ( 'NONE', #21326, 0.3066721922917531873, 0.5845243560369969282 ) ;
#11386=EDGE_LOOP ( 'NONE', ( #9114, #13912, #4514, #14867 ) ) ;
#11407=CARTESIAN_POINT ( 'NONE',  ( 0.3722026523000413478, 4.558167867734008572E-17, -0.2204724409448818867 ) ) ;
#11408=DIRECTION ( 'NONE',  ( 1.000000000000000000, 0.000000000000000000, 0.000000000000000000 ) ) ;
#11409=CARTESIAN_POINT ( 'NONE',  ( 0.4010740433761567081, 4.911740434416970370E-17, -0.2342519685039370358 ) ) ;
#11414=ORIENTED_EDGE ( 'NONE', *, *, #19334, .T. ) ;
#11420=CARTESIAN_POINT ( 'NONE',  ( 0.5118110236220472231, 6.267877318470705905E-17, -0.2618110236220472231 ) ) ;
#11445=DIRECTION ( 'NONE',  ( 0.000000000000000000, 0.000000000000000000, -1.000000000000000000 ) ) ;
#11468=TOROIDAL_SURFACE ( 'NONE', #6095, 0.4980314960629921295, 0.01377952755905511792 ) ;
#11547=DIRECTION ( 'NONE',  ( 0.000000000000000000, 0.000000000000000000, -1.000000000000000000 ) ) ;
#11570=DIRECTION ( 'NONE',  ( -1.000000000000000000, 0.000000000000000000, 0.000000000000000000 ) ) ;
#11572=AXIS2_PLACEMENT_3D ( 'NONE', #26391, #4922, #434 ) ;
#11578=UNCERTAINTY_MEASURE_WITH_UNIT (LENGTH_MEASURE( 1.000000000000000082E-05 ), #21537, 'distance_accuracy_value', 'NONE') ;
#11588=AXIS2_PLACEMENT_3D ( 'NONE', #5229, #3665, #7923 ) ;
#11590=CARTESIAN_POINT ( 'NONE',  ( 0.2952755905511810774, -3.755651186670777132E-17, -0.07578740157480315376 ) ) ;
#11612=DIRECTION ( 'NONE',  ( 0.000000000000000000, 0.000000000000000000, -1.000000000000000000 ) ) ;
#11619=AXIS2_PLACEMENT_3D ( 'NONE', #2132, #19222, #4658 ) ;
#11645=CIRCLE ( 'NONE', #2180, 0.3294268239956709143 ) ;
#11651=AXIS2_PLACEMENT_3D ( 'NONE', #14438, #18784, #23191 ) ;
#11656=DIRECTION ( 'NONE',  ( 0.000000000000000000, 0.000000000000000000, 1.000000000000000000 ) ) ;
#11696=ORIENTED_EDGE ( 'NONE', *, *, #20438, .T. ) ;
#11738=FACE_OUTER_BOUND ( 'NONE', #8717, .T. ) ;
#11792=ORIENTED_EDGE ( 'NONE', *, *, #25585, .T. ) ;
#11888=CARTESIAN_POINT ( 'NONE',  ( -0.3722026523000413478, 0.000000000000000000, -0.05856299212598425896 ) ) ;
#11899=DIRECTION ( 'NONE',  ( 0.000000000000000000, 0.000000000000000000, -1.000000000000000000 ) ) ;
#11998=CARTESIAN_POINT ( 'NONE',  ( 0.3458446900868161200, 4.235375927169277411E-17, -0.2204724409448818867 ) ) ;
#12015=ORIENTED_EDGE ( 'NONE', *, *, #21562, .T. ) ;
#12074=CIRCLE ( 'NONE', #26917, 0.01377952755905510404 ) ;
#12118=VERTEX_POINT ( 'NONE', #10476 ) ;
#12154=ORIENTED_EDGE ( 'NONE', *, *, #862, .F. ) ;
#12197=CARTESIAN_POINT ( 'NONE',  ( 0.000000000000000000, 0.000000000000000000, -6.283251968503937502E-17 ) ) ;
#12209=ORIENTED_EDGE ( 'NONE', *, *, #8880, .T. ) ;
#12232=ORIENTED_EDGE ( 'NONE', *, *, #4565, .T. ) ;
#12258=DIRECTION ( 'NONE',  ( 0.000000000000000000, 0.000000000000000000, -1.000000000000000000 ) ) ;
#12294=FACE_BOUND ( 'NONE', #520, .T. ) ;
#12296=DIMENSIONAL_EXPONENTS ( 1.000000000000000000, 0.000000000000000000, 0.000000000000000000, 0.000000000000000000, 0.000000000000000000, 0.000000000000000000, 0.000000000000000000 ) ;
#12345=AXIS2_PLACEMENT_3D ( 'NONE', #22887, #16381, #19049 ) ;
#12359=ORIENTED_EDGE ( 'NONE', *, *, #13812, .T. ) ;
#12394=DIRECTION ( 'NONE',  ( 0.000000000000000000, 0.000000000000000000, 1.000000000000000000 ) ) ;
#12427=CARTESIAN_POINT ( 'NONE',  ( -0.3722026523000413478, 0.000000000000000000, -0.05511811023622047168 ) ) ;
#12432=DIRECTION ( 'NONE',  ( -1.000000000000000000, 0.000000000000000000, 0.000000000000000000 ) ) ;
#12441=ORIENTED_EDGE ( 'NONE', *, *, #11215, .T. ) ;
#12448=DIRECTION ( 'NONE',  ( -1.000000000000000000, 0.000000000000000000, 0.000000000000000000 ) ) ;
#12472=DIRECTION ( 'NONE',  ( 0.000000000000000000, 0.000000000000000000, 1.000000000000000000 ) ) ;
#12498=EDGE_LOOP ( 'NONE', ( #25731, #4495, #5923, #4131 ) ) ;
#12531=COLOUR_RGB ( '', 0.09019608, 0.27058824, 0.51372549) ;
#12548=AXIS2_PLACEMENT_3D ( 'NONE', #4790, #13281, #21905 ) ;
#12574=DIRECTION ( 'NONE',  ( 0.000000000000000000, 0.000000000000000000, -1.000000000000000000 ) ) ;
#12689=DIRECTION ( 'NONE',  ( 1.000000000000000000, 0.000000000000000000, 0.000000000000000000 ) ) ;
#12740=VECTOR ( 'NONE', #19778, 39.37007874015748854 ) ;
#12825=VERTEX_POINT ( 'NONE', #18922 ) ;
#12854=ADVANCED_FACE ( 'NONE', ( #3959, #16291 ), #21195, .T. ) ;
#12880=ORIENTED_EDGE ( 'NONE', *, *, #20059, .F. ) ;
#12938=EDGE_CURVE ( 'NONE', #12118, #18288, #4938, .T. ) ;
#12952=ORIENTED_EDGE ( 'NONE', *, *, #5362, .F. ) ;
#12971=( GEOMETRIC_REPRESENTATION_CONTEXT ( 3 ) GLOBAL_UNCERTAINTY_ASSIGNED_CONTEXT ( ( #11578 ) ) GLOBAL_UNIT_ASSIGNED_CONTEXT ( ( #21537, #19558, #21813 ) ) REPRESENTATION_CONTEXT ( 'NONE', 'WORKASPACE' ) ) ;
#12996=DIRECTION ( 'NONE',  ( -1.000000000000000000, 0.000000000000000000, 0.000000000000000000 ) ) ;
#13009=DIRECTION ( 'NONE',  ( -1.000000000000000000, 0.000000000000000000, 0.000000000000000000 ) ) ;
#13010=CARTESIAN_POINT ( 'NONE',  ( 0.000000000000000000, 0.000000000000000000, -0.2204724409448818867 ) ) ;
#13031=EDGE_LOOP ( 'NONE', ( #9379, #18411, #25686, #6258 ) ) ;
#13045=DIMENSIONAL_EXPONENTS ( 1.000000000000000000, 0.000000000000000000, 0.000000000000000000, 0.000000000000000000, 0.000000000000000000, 0.000000000000000000, 0.000000000000000000 ) ;
#13078=VERTEX_POINT ( 'NONE', #15216 ) ;
#13138=DIRECTION ( 'NONE',  ( 0.000000000000000000, 0.000000000000000000, -1.000000000000000000 ) ) ;
#13156=CIRCLE ( 'NONE', #993, 0.5118110236220472231 ) ;
#13179=ORIENTED_EDGE ( 'NONE', *, *, #13927, .T. ) ;
#13190=CARTESIAN_POINT ( 'NONE',  ( -0.4010740433761567081, 0.000000000000000000, -0.2480314960629921295 ) ) ;
#13222=CIRCLE ( 'NONE', #4653, 0.5118110236220472231 ) ;
#13239=ORIENTED_EDGE ( 'NONE', *, *, #18218, .T. ) ;
#13254=CARTESIAN_POINT ( 'NONE',  ( 0.000000000000000000, 0.000000000000000000, -0.2204724409448818867 ) ) ;
#13255=DIRECTION ( 'NONE',  ( -1.000000000000000000, 0.000000000000000000, 0.000000000000000000 ) ) ;
#13277=DIRECTION ( 'NONE',  ( -0.000000000000000000, -1.000000000000000000, -0.000000000000000000 ) ) ;
#13281=DIRECTION ( 'NONE',  ( -0.000000000000000000, -1.000000000000000000, -0.000000000000000000 ) ) ;
#13360=ORIENTED_EDGE ( 'NONE', *, *, #6046, .F. ) ;
#13382=ORIENTED_EDGE ( 'NONE', *, *, #1096, .F. ) ;
#13426=CARTESIAN_POINT ( 'NONE',  ( 0.000000000000000000, 0.000000000000000000, -0.1309055118110236116 ) ) ;
#13460=TOROIDAL_SURFACE ( 'NONE', #19348, 0.4980314960629921295, 0.01377952755905511792 ) ;
#13526=ADVANCED_FACE ( 'NONE', ( #14888 ), #5972, .T. ) ;
#13530=( NAMED_UNIT ( * ) SI_UNIT ( $, .STERADIAN. ) SOLID_ANGLE_UNIT ( ) ) ;
#13532=EDGE_LOOP ( 'NONE', ( #27664, #11414, #10546, #23478 ) ) ;
#13551=ADVANCED_FACE ( 'NONE', ( #15690 ), #7340, .F. ) ;
#13552=ADVANCED_FACE ( 'NONE', ( #4543 ), #9042, .T. ) ;
#13554=DIRECTION ( 'NONE',  ( 0.000000000000000000, 0.000000000000000000, -1.000000000000000000 ) ) ;
#13575=CIRCLE ( 'NONE', #10419, 0.4010740433761567081 ) ;
#13603=CARTESIAN_POINT ( 'NONE',  ( 0.000000000000000000, 0.000000000000000000, -0.2342519685039370358 ) ) ;
#13662=DIRECTION ( 'NONE',  ( 0.000000000000000000, 0.000000000000000000, -1.000000000000000000 ) ) ;
#13682=ORIENTED_EDGE ( 'NONE', *, *, #1071, .T. ) ;
#13696=DIRECTION ( 'NONE',  ( 0.000000000000000000, 0.000000000000000000, -1.000000000000000000 ) ) ;
#13702=VECTOR ( 'NONE', #11445, 39.37007874015748143 ) ;
#13703=ADVANCED_FACE ( 'NONE', ( #26148 ), #10054, .T. ) ;
#13704=ORIENTED_EDGE ( 'NONE', *, *, #17477, .F. ) ;
#13709=DIRECTION ( 'NONE',  ( 0.000000000000000000, 0.000000000000000000, -1.000000000000000000 ) ) ;
#13812=EDGE_CURVE ( 'NONE', #9956, #24011, #10522, .T. ) ;
#13845=CARTESIAN_POINT ( 'NONE',  ( 0.000000000000000000, 0.000000000000000000, -6.010066929133858501E-17 ) ) ;
#13855=AXIS2_PLACEMENT_3D ( 'NONE', #8267, #6167, #14793 ) ;
#13862=EDGE_CURVE ( 'NONE', #19453, #24685, #20897, .T. ) ;
#13886=EDGE_LOOP ( 'NONE', ( #26659, #15035, #10177, #14665 ) ) ;
#13910=LINE ( 'NONE', #3156, #10790 ) ;
#13912=ORIENTED_EDGE ( 'NONE', *, *, #1001, .F. ) ;
#13927=EDGE_CURVE ( 'NONE', #26909, #19035, #13222, .T. ) ;
#13982=CIRCLE ( 'NONE', #24325, 0.3722026523000413478 ) ;
#14002=VERTEX_POINT ( 'NONE', #12427 ) ;
#14019=EDGE_CURVE ( 'NONE', #10626, #17531, #10541, .T. ) ;
#14024=EDGE_LOOP ( 'NONE', ( #13239, #18923, #23835, #13704 ) ) ;
#14025=CARTESIAN_POINT ( 'NONE',  ( 0.3584231247409862542, 4.473792596139210520E-17, -0.04133858267716535029 ) ) ;
#14030=LINE ( 'NONE', #24205, #8379 ) ;
#14068=ORIENTED_EDGE ( 'NONE', *, *, #22966, .F. ) ;
#14106=ADVANCED_FACE ( 'NONE', ( #19340 ), #630, .F. ) ;
#14116=ORIENTED_EDGE ( 'NONE', *, *, #5362, .T. ) ;
#14117=AXIS2_PLACEMENT_3D ( 'NONE', #8136, #1765, #4174 ) ;
#14126=DIRECTION ( 'NONE',  ( 1.000000000000000000, 0.000000000000000000, 0.000000000000000000 ) ) ;
#14143=DIRECTION ( 'NONE',  ( -1.000000000000000000, 0.000000000000000000, 0.000000000000000000 ) ) ;
#14147=DIRECTION ( 'NONE',  ( -1.000000000000000000, 0.000000000000000000, 0.000000000000000000 ) ) ;
#14238=DIRECTION ( 'NONE',  ( -1.224646799147353207E-16, 1.000000000000000000, 0.000000000000000000 ) ) ;
#14277=DIRECTION ( 'NONE',  ( 1.000000000000000000, 0.000000000000000000, 0.000000000000000000 ) ) ;
#14301=LINE ( 'NONE', #10323, #22322 ) ;
#14311=AXIS2_PLACEMENT_3D ( 'NONE', #5833, #1436, #13009 ) ;
#14330=VECTOR ( 'NONE', #20120, 39.37007874015748143 ) ;
#14356=AXIS2_PLACEMENT_3D ( 'NONE', #9795, #5426, #10487 ) ;
#14403=CIRCLE ( 'NONE', #2199, 0.4842519685039370358 ) ;
#14412=ORIENTED_EDGE ( 'NONE', *, *, #11215, .F. ) ;
#14436=AXIS2_PLACEMENT_3D ( 'NONE', #11367, #2868, #23957 ) ;
#14438=CARTESIAN_POINT ( 'NONE',  ( -0.4426630059400472605, 0.000000000000000000, -0.2480314960629921295 ) ) ;
#14470=CARTESIAN_POINT ( 'NONE',  ( 0.3584231247409862542, 4.389417324544413085E-17, -0.05511811023622047168 ) ) ;
#14472=EDGE_CURVE ( 'NONE', #20206, #24622, #24997, .T. ) ;
#14490=PRODUCT_DEFINITION_CONTEXT ( 'detailed design', #20452, 'design' ) ;
#14592=VERTEX_POINT ( 'NONE', #14025 ) ;
#14622=PLANE ( 'NONE',  #19225 ) ;
#14665=ORIENTED_EDGE ( 'NONE', *, *, #23833, .F. ) ;
#14668=AXIS2_PLACEMENT_3D ( 'NONE', #23179, #1690, #12432 ) ;
#14700=CONICAL_SURFACE ( 'NONE', #684, 0.3224687058348476576, 0.8056700744428512140 ) ;
#14739=EDGE_LOOP ( 'NONE', ( #14782, #4917, #18187, #19771 ) ) ;
#14771=EDGE_LOOP ( 'NONE', ( #7573, #1521 ) ) ;
#14782=ORIENTED_EDGE ( 'NONE', *, *, #751, .T. ) ;
#14793=DIRECTION ( 'NONE',  ( -1.000000000000000000, 0.000000000000000000, 0.000000000000000000 ) ) ;
#14867=ORIENTED_EDGE ( 'NONE', *, *, #4152, .T. ) ;
#14871=EDGE_CURVE ( 'NONE', #19035, #17310, #24029, .T. ) ;
#14875=DIRECTION ( 'NONE',  ( 0.000000000000000000, 0.000000000000000000, -1.000000000000000000 ) ) ;
#14887=EDGE_LOOP ( 'NONE', ( #2606, #26193, #8035, #2335 ) ) ;
#14888=FACE_OUTER_BOUND ( 'NONE', #1940, .T. ) ;
#14901=CARTESIAN_POINT ( 'NONE',  ( 0.4685039370078740717, 5.737518468446261360E-17, -6.283251968503937502E-17 ) ) ;
#14932=EDGE_CURVE ( 'NONE', #8592, #9665, #24302, .T. ) ;
#14938=CARTESIAN_POINT ( 'NONE',  ( 0.000000000000000000, 0.000000000000000000, -0.006889763779527558960 ) ) ;
#15035=ORIENTED_EDGE ( 'NONE', *, *, #21568, .T. ) ;
#15089=CIRCLE ( 'NONE', #15974, 0.4010740433761567081 ) ;
#15092=PRODUCT_CONTEXT ( 'NONE', #17041, 'mechanical' ) ;
#15143=DIRECTION ( 'NONE',  ( 0.000000000000000000, 0.000000000000000000, -1.000000000000000000 ) ) ;
#15146=DIRECTION ( 'NONE',  ( -1.000000000000000000, 0.000000000000000000, 0.000000000000000000 ) ) ;
#15169=AXIS2_PLACEMENT_3D ( 'NONE', #17784, #13138, #11570 ) ;
#15216=CARTESIAN_POINT ( 'NONE',  ( -0.3332647802741406373, -9.151579316449505861E-28, -0.1692378991623492424 ) ) ;
#15223=CARTESIAN_POINT ( 'NONE',  ( -0.3126261861395013275, 0.000000000000000000, -0.1464516454673935042 ) ) ;
#15255=ADVANCED_FACE ( 'NONE', ( #23470 ), #10579, .T. ) ;
#15261=LINE ( 'NONE', #8341, #4698 ) ;
#15383=DIRECTION ( 'NONE',  ( -1.000000000000000000, 0.000000000000000000, 0.000000000000000000 ) ) ;
#15459=EDGE_CURVE ( 'NONE', #26519, #23791, #18241, .T. ) ;
#15485=AXIS2_PLACEMENT_3D ( 'NONE', #10329, #23496, #21501 ) ;
#15553=DIRECTION ( 'NONE',  ( -1.000000000000000000, 0.000000000000000000, 0.000000000000000000 ) ) ;
#15558=CARTESIAN_POINT ( 'NONE',  ( 0.3180687940157840843, -3.895219305000888202E-17, -0.04133858267716535029 ) ) ;
#15560=CIRCLE ( 'NONE', #5627, 0.4685039370078740717 ) ;
#15566=DIRECTION ( 'NONE',  ( -1.000000000000000000, 0.000000000000000000, 0.000000000000000000 ) ) ;
#15569=CIRCLE ( 'NONE', #7435, 0.3332647802741406373 ) ;
#15572=ADVANCED_FACE ( 'NONE', ( #4709 ), #14700, .F. ) ;
#15679=DIRECTION ( 'NONE',  ( -1.000000000000000000, 0.000000000000000000, 0.000000000000000000 ) ) ;
#15690=FACE_OUTER_BOUND ( 'NONE', #1475, .T. ) ;
#15719=EDGE_CURVE ( 'NONE', #9665, #3782, #265, .T. ) ;
#15810=CARTESIAN_POINT ( 'NONE',  ( 0.000000000000000000, 0.000000000000000000, -0.05856299212598425896 ) ) ;
#15823=CARTESIAN_POINT ( 'NONE',  ( 0.000000000000000000, 0.000000000000000000, -0.2755905511811023723 ) ) ;
#15884=EDGE_CURVE ( 'NONE', #26909, #19062, #14030, .T. ) ;
#15941=AXIS2_PLACEMENT_3D ( 'NONE', #19947, #24733, #3113 ) ;
#15944=ORIENTED_EDGE ( 'NONE', *, *, #21568, .F. ) ;
#15950=AXIS2_PLACEMENT_3D ( 'NONE', #26377, #41, #8873 ) ;
#15953=DIRECTION ( 'NONE',  ( 0.000000000000000000, -1.000000000000000000, 0.000000000000000000 ) ) ;
#15956=DIRECTION ( 'NONE',  ( 0.000000000000000000, 0.000000000000000000, 1.000000000000000000 ) ) ;
#15963=CIRCLE ( 'NONE', #11006, 0.3584231247409862542 ) ;
#15974=AXIS2_PLACEMENT_3D ( 'NONE', #17405, #6955, #6817 ) ;
#15976=ORIENTED_EDGE ( 'NONE', *, *, #6046, .T. ) ;
#16025=DIRECTION ( 'NONE',  ( -1.000000000000000000, -1.224646799147356165E-16, 0.000000000000000000 ) ) ;
#16177=TOROIDAL_SURFACE ( 'NONE', #6698, 0.4980314960629921295, 0.01377952755905511792 ) ;
#16254=DIRECTION ( 'NONE',  ( -1.000000000000000000, 0.000000000000000000, 0.000000000000000000 ) ) ;
#16274=DIRECTION ( 'NONE',  ( 0.000000000000000000, 0.000000000000000000, -1.000000000000000000 ) ) ;
#16291=FACE_OUTER_BOUND ( 'NONE', #9157, .T. ) ;
#16340=CARTESIAN_POINT ( 'NONE',  ( 0.4685039370078740717, 5.737518468446261360E-17, -0.006889763779527558960 ) ) ;
#16381=DIRECTION ( 'NONE',  ( 0.000000000000000000, 0.000000000000000000, -1.000000000000000000 ) ) ;
#16396=ADVANCED_FACE ( 'NONE', ( #11738 ), #27421, .T. ) ;
#16461=VERTEX_POINT ( 'NONE', #21207 ) ;
#16481=CARTESIAN_POINT ( 'NONE',  ( -0.4842519685039370358, 0.000000000000000000, -0.1309055118110236116 ) ) ;
#16513=AXIS2_PLACEMENT_3D ( 'NONE', #16525, #23190, #14147 ) ;
#16514=DIRECTION ( 'NONE',  ( -1.000000000000000000, 0.000000000000000000, 0.000000000000000000 ) ) ;
#16515=CARTESIAN_POINT ( 'NONE',  ( 0.3722026523000413478, 4.558167867734008572E-17, -0.05511811023622047168 ) ) ;
#16525=CARTESIAN_POINT ( 'NONE',  ( 0.000000000000000000, 0.000000000000000000, -0.1377952755905511861 ) ) ;
#16529=CARTESIAN_POINT ( 'NONE',  ( 0.3198827364362346048, 3.917433692791311553E-17, -0.1725236688546921415 ) ) ;
#16546=( LENGTH_UNIT ( ) NAMED_UNIT ( * ) SI_UNIT ( $, .METRE. ) ) ;
#16639=EDGE_CURVE ( 'NONE', #9956, #19035, #26595, .T. ) ;
#16645=VECTOR ( 'NONE', #13662, 39.37007874015748143 ) ;
#16708=EDGE_CURVE ( 'NONE', #24827, #11368, #7209, .T. ) ;
#16714=DIRECTION ( 'NONE',  ( -1.000000000000000000, -1.224646799147356165E-16, 0.000000000000000000 ) ) ;
#16731=ORIENTED_EDGE ( 'NONE', *, *, #20438, .F. ) ;
#16787=ADVANCED_FACE ( 'NONE', ( #9570 ), #10824, .F. ) ;
#16794=ORIENTED_EDGE ( 'NONE', *, *, #6993, .F. ) ;
#16894=AXIS2_PLACEMENT_3D ( 'NONE', #27741, #1736, #23223 ) ;
#16942=EDGE_LOOP ( 'NONE', ( #27654, #3264 ) ) ;
#16949=DIRECTION ( 'NONE',  ( 0.000000000000000000, 0.000000000000000000, 1.000000000000000000 ) ) ;
#16976=CIRCLE ( 'NONE', #26903, 0.3294268239956709143 ) ;
#17012=AXIS2_PLACEMENT_3D ( 'NONE', #17307, #499, #19976 ) ;
#17038=FACE_OUTER_BOUND ( 'NONE', #23186, .T. ) ;
#17041=APPLICATION_CONTEXT ( 'automotive_design' ) ;
#17084=DIRECTION ( 'NONE',  ( 1.000000000000000000, 0.000000000000000000, 0.000000000000000000 ) ) ;
#17101=EDGE_CURVE ( 'NONE', #26519, #8592, #23087, .T. ) ;
#17149=DIRECTION ( 'NONE',  ( -1.000000000000000000, 0.000000000000000000, 0.000000000000000000 ) ) ;
#17183=EDGE_CURVE ( 'NONE', #1325, #8592, #6346, .T. ) ;
#17232=ORIENTED_EDGE ( 'NONE', *, *, #675, .F. ) ;
#17243=ORIENTED_EDGE ( 'NONE', *, *, #81, .F. ) ;
#17300=AXIS2_PLACEMENT_3D ( 'NONE', #18168, #27105, #26661 ) ;
#17307=CARTESIAN_POINT ( 'NONE',  ( 0.000000000000000000, 0.000000000000000000, -0.1309055118110236116 ) ) ;
#17310=VERTEX_POINT ( 'NONE', #2163 ) ;
#17317=DIRECTION ( 'NONE',  ( 1.000000000000000000, 0.000000000000000000, 0.000000000000000000 ) ) ;
#17398=CARTESIAN_POINT ( 'NONE',  ( 0.3224687058348476576, 3.949102684258356242E-17, -0.1559029880880275776 ) ) ;
#17405=CARTESIAN_POINT ( 'NONE',  ( 0.000000000000000000, 0.000000000000000000, -0.2342519685039370358 ) ) ;
#17470=ORIENTED_EDGE ( 'NONE', *, *, #4185, .F. ) ;
#17477=EDGE_CURVE ( 'NONE', #17310, #24685, #23377, .T. ) ;
#17516=EDGE_CURVE ( 'NONE', #5769, #22371, #25171, .T. ) ;
#17531=VERTEX_POINT ( 'NONE', #15558 ) ;
#17569=CIRCLE ( 'NONE', #26554, 0.01377952755905510404 ) ;
#17583=AXIS2_PLACEMENT_3D ( 'NONE', #18298, #5324, #9543 ) ;
#17592=EDGE_CURVE ( 'NONE', #9997, #25216, #25630, .T. ) ;
#17626=FACE_OUTER_BOUND ( 'NONE', #13031, .T. ) ;
#17637=LENGTH_MEASURE_WITH_UNIT ( LENGTH_MEASURE( 0.02539999999999999897 ), #24002 ) ;
#17638=ORIENTED_EDGE ( 'NONE', *, *, #16708, .T. ) ;
#17673=EDGE_LOOP ( 'NONE', ( #4672, #12209, #4960, #4076 ) ) ;
#17710=EDGE_LOOP ( 'NONE', ( #19378, #12441, #19929, #17243 ) ) ;
#17735=DIRECTION ( 'NONE',  ( 0.000000000000000000, 0.000000000000000000, -1.000000000000000000 ) ) ;
#17784=CARTESIAN_POINT ( 'NONE',  ( 0.000000000000000000, 0.000000000000000000, -0.1756889763779527769 ) ) ;
#17816=CARTESIAN_POINT ( 'NONE',  ( 0.4980314960629921295, 6.099126775281109802E-17, -0.01377952755905511792 ) ) ;
#17841=FACE_OUTER_BOUND ( 'NONE', #14024, .T. ) ;
#17860=AXIS2_PLACEMENT_3D ( 'NONE', #14938, #19143, #21413 ) ;
#17877=DIRECTION ( 'NONE',  ( -1.000000000000000000, 0.000000000000000000, 0.000000000000000000 ) ) ;
#17887=EDGE_CURVE ( 'NONE', #3782, #12825, #23165, .T. ) ;
#17893=EDGE_LOOP ( 'NONE', ( #18131, #23583 ) ) ;
#17926=DIRECTION ( 'NONE',  ( -1.000000000000000000, 0.000000000000000000, 0.000000000000000000 ) ) ;
#18013=CARTESIAN_POINT ( 'NONE',  ( 0.000000000000000000, 0.000000000000000000, -0.2755905511811023723 ) ) ;
#18082=DIRECTION ( 'NONE',  ( 0.000000000000000000, 0.000000000000000000, 1.000000000000000000 ) ) ;
#18131=ORIENTED_EDGE ( 'NONE', *, *, #14019, .T. ) ;
#18154=ADVANCED_FACE ( 'NONE', ( #19886 ), #16177, .T. ) ;
#18168=CARTESIAN_POINT ( 'NONE',  ( 0.000000000000000000, 0.000000000000000000, -0.1111195235210984261 ) ) ;
#18170=CLOSED_SHELL ( 'NONE', ( #3969, #15255, #3574, #19135, #14106, #6549, #6081, #20940, #26660, #18154, #27265, #22637, #16787, #10845, #13526, #26597, #12854, #27332, #20536, #26158, #23647, #9017, #6298, #9983, #21250, #24871, #6838, #21094, #22058, #15572, #13551, #23779, #16396, #20024, #13703, #13552, #24739, #2415 ) ) ;
#18187=ORIENTED_EDGE ( 'NONE', *, *, #6583, .F. ) ;
#18218=EDGE_CURVE ( 'NONE', #17310, #19062, #1292, .T. ) ;
#18241=CIRCLE ( 'NONE', #2901, 0.2952755905511810774 ) ;
#18288=VERTEX_POINT ( 'NONE', #1780 ) ;
#18298=CARTESIAN_POINT ( 'NONE',  ( 0.000000000000000000, 0.000000000000000000, -0.1111195235210984261 ) ) ;
#18304=DIRECTION ( 'NONE',  ( -1.000000000000000000, 0.000000000000000000, 0.000000000000000000 ) ) ;
#18411=ORIENTED_EDGE ( 'NONE', *, *, #20059, .T. ) ;
#18427=TOROIDAL_SURFACE ( 'NONE', #22958, 0.3872945158171015589, 0.01377952755905511792 ) ;
#18436=CARTESIAN_POINT ( 'NONE',  ( 0.3722026523000413478, 4.558167867734008572E-17, -0.1033464566929133965 ) ) ;
#18455=ORIENTED_EDGE ( 'NONE', *, *, #1001, .T. ) ;
#18466=EDGE_LOOP ( 'NONE', ( #8355, #6647, #4243, #5808 ) ) ;
#18527=FACE_OUTER_BOUND ( 'NONE', #10006, .T. ) ;
#18562=FACE_OUTER_BOUND ( 'NONE', #14739, .T. ) ;
#18572=AXIS2_PLACEMENT_3D ( 'NONE', #24894, #12574, #19060 ) ;
#18638=AXIS2_PLACEMENT_3D ( 'NONE', #25276, #7772, #14126 ) ;
#18667=CARTESIAN_POINT ( 'NONE',  ( 0.4010740433761567081, 4.911740434416970370E-17, -0.2342519685039370358 ) ) ;
#18716=CYLINDRICAL_SURFACE ( 'NONE', #17860, 0.4685039370078740717 ) ;
#18784=DIRECTION ( 'NONE',  ( 0.000000000000000000, 0.000000000000000000, 1.000000000000000000 ) ) ;
#18812=VERTEX_POINT ( 'NONE', #3414 ) ;
#18864=DIRECTION ( 'NONE',  ( 0.000000000000000000, 0.000000000000000000, -1.000000000000000000 ) ) ;
#18877=DIRECTION ( 'NONE',  ( -1.000000000000000000, 0.000000000000000000, 0.000000000000000000 ) ) ;
#18885=EDGE_LOOP ( 'NONE', ( #22721, #19369, #5475, #12880 ) ) ;
#18922=CARTESIAN_POINT ( 'NONE',  ( 0.3593781546376668135, 4.401113067605012182E-17, -0.2755905511811023723 ) ) ;
#18923=ORIENTED_EDGE ( 'NONE', *, *, #20993, .T. ) ;
#18928=ORIENTED_EDGE ( 'NONE', *, *, #14932, .T. ) ;
#18935=DIRECTION ( 'NONE',  ( 0.000000000000000000, 0.000000000000000000, -1.000000000000000000 ) ) ;
#18947=AXIS2_PLACEMENT_3D ( 'NONE', #15810, #26821, #15679 ) ;
#18952=DIRECTION ( 'NONE',  ( -1.000000000000000000, 0.000000000000000000, 0.000000000000000000 ) ) ;
#19035=VERTEX_POINT ( 'NONE', #10803 ) ;
#19043=DIRECTION ( 'NONE',  ( 0.000000000000000000, 0.000000000000000000, 1.000000000000000000 ) ) ;
#19049=DIRECTION ( 'NONE',  ( -1.000000000000000000, 0.000000000000000000, 0.000000000000000000 ) ) ;
#19060=DIRECTION ( 'NONE',  ( 0.000000000000000000, -1.000000000000000000, 0.000000000000000000 ) ) ;
#19062=VERTEX_POINT ( 'NONE', #11420 ) ;
#19073=EDGE_LOOP ( 'NONE', ( #17232, #1023, #10974, #3860 ) ) ;
#19094=CIRCLE ( 'NONE', #22704, 0.4842519685039370358 ) ;
#19120=CARTESIAN_POINT ( 'NONE',  ( 0.000000000000000000, 0.000000000000000000, -0.05511811023622047168 ) ) ;
#19135=ADVANCED_FACE ( 'NONE', ( #25992 ), #22160, .T. ) ;
#19136=CIRCLE ( 'NONE', #16894, 0.3722026523000413478 ) ;
#19143=DIRECTION ( 'NONE',  ( 0.000000000000000000, 0.000000000000000000, -1.000000000000000000 ) ) ;
#19172=ORIENTED_EDGE ( 'NONE', *, *, #9105, .T. ) ;
#19191=DIRECTION ( 'NONE',  ( 0.000000000000000000, 0.000000000000000000, 1.000000000000000000 ) ) ;
#19222=DIRECTION ( 'NONE',  ( -0.000000000000000000, -1.000000000000000000, -0.000000000000000000 ) ) ;
#19225=AXIS2_PLACEMENT_3D ( 'NONE', #1322, #25044, #27450 ) ;
#19235=EDGE_CURVE ( 'NONE', #1325, #26728, #1842, .T. ) ;
#19274=FILL_AREA_STYLE_COLOUR ( '', #12531 ) ;
#19282=ORIENTED_EDGE ( 'NONE', *, *, #21913, .T. ) ;
#19284=ORIENTED_EDGE ( 'NONE', *, *, #7598, .T. ) ;
#19322=ORIENTED_EDGE ( 'NONE', *, *, #27699, .T. ) ;
#19334=EDGE_CURVE ( 'NONE', #7273, #25216, #10693, .T. ) ;
#19340=FACE_OUTER_BOUND ( 'NONE', #9149, .T. ) ;
#19348=AXIS2_PLACEMENT_3D ( 'NONE', #2191, #11089, #117 ) ;
#19369=ORIENTED_EDGE ( 'NONE', *, *, #17183, .F. ) ;
#19378=ORIENTED_EDGE ( 'NONE', *, *, #296, .T. ) ;
#19390=DIRECTION ( 'NONE',  ( -1.224646799147353207E-16, 1.000000000000000000, 0.000000000000000000 ) ) ;
#19396=CARTESIAN_POINT ( 'NONE',  ( -0.4901574803149605919, 0.000000000000000000, -6.034492125984251821E-17 ) ) ;
#19453=VERTEX_POINT ( 'NONE', #22257 ) ;
#19472=CARTESIAN_POINT ( 'NONE',  ( -0.2952755905511810774, 0.000000000000000000, -0.07578740157480315376 ) ) ;
#19558=( NAMED_UNIT ( * ) PLANE_ANGLE_UNIT ( ) SI_UNIT ( $, .RADIAN. ) ) ;
#19559=CIRCLE ( 'NONE', #27690, 0.01377952755905511965 ) ;
#19627=CIRCLE ( 'NONE', #20520, 0.4010740433761567081 ) ;
#19670=ORIENTED_EDGE ( 'NONE', *, *, #81, .T. ) ;
#19679=DIRECTION ( 'NONE',  ( 0.000000000000000000, 0.000000000000000000, 1.000000000000000000 ) ) ;
#19693=DIRECTION ( 'NONE',  ( -1.000000000000000000, 0.000000000000000000, 0.000000000000000000 ) ) ;
#19696=AXIS2_PLACEMENT_3D ( 'NONE', #27740, #10060, #1451 ) ;
#19771=ORIENTED_EDGE ( 'NONE', *, *, #17592, .F. ) ;
#19778=DIRECTION ( 'NONE',  ( -0.2384530002628495460, 0.000000000000000000, -0.9711540385879292581 ) ) ;
#19819=DIRECTION ( 'NONE',  ( 0.000000000000000000, 0.000000000000000000, -1.000000000000000000 ) ) ;
#19827=SURFACE_SIDE_STYLE ('',( #10799 ) ) ;
#19833=ORIENTED_EDGE ( 'NONE', *, *, #25383, .F. ) ;
#19851=DIRECTION ( 'NONE',  ( -1.000000000000000000, 0.000000000000000000, 0.000000000000000000 ) ) ;
#19886=FACE_OUTER_BOUND ( 'NONE', #4073, .T. ) ;
#19887=CARTESIAN_POINT ( 'NONE',  ( 0.000000000000000000, 0.000000000000000000, -0.01377952755905511792 ) ) ;
#19902=EDGE_CURVE ( 'NONE', #4205, #3117, #8402, .T. ) ;
#19917=CARTESIAN_POINT ( 'NONE',  ( 0.000000000000000000, 0.000000000000000000, -0.05856299212598425896 ) ) ;
#19929=ORIENTED_EDGE ( 'NONE', *, *, #23570, .T. ) ;
#19947=CARTESIAN_POINT ( 'NONE',  ( 0.000000000000000000, 0.000000000000000000, -0.006889763779527558960 ) ) ;
#19976=DIRECTION ( 'NONE',  ( -1.000000000000000000, 0.000000000000000000, 0.000000000000000000 ) ) ;
#20024=ADVANCED_FACE ( 'NONE', ( #23372, #18527 ), #14622, .T. ) ;
#20027=DIRECTION ( 'NONE',  ( 0.000000000000000000, 0.000000000000000000, -1.000000000000000000 ) ) ;
#20059=EDGE_CURVE ( 'NONE', #9665, #26728, #16976, .T. ) ;
#20062=AXIS2_PLACEMENT_3D ( 'NONE', #21336, #25705, #25284 ) ;
#20120=DIRECTION ( 'NONE',  ( 0.000000000000000000, 0.000000000000000000, -1.000000000000000000 ) ) ;
#20142=ORIENTED_EDGE ( 'NONE', *, *, #1850, .T. ) ;
#20194=EDGE_LOOP ( 'NONE', ( #2529, #20773 ) ) ;
#20206=VERTEX_POINT ( 'NONE', #14901 ) ;
#20233=CARTESIAN_POINT ( 'NONE',  ( 0.000000000000000000, 0.000000000000000000, -6.283251968503937502E-17 ) ) ;
#20236=AXIS2_PLACEMENT_3D ( 'NONE', #13254, #20027, #11408 ) ;
#20248=ORIENTED_EDGE ( 'NONE', *, *, #9105, .F. ) ;
#20254=DIRECTION ( 'NONE',  ( -1.000000000000000000, 0.000000000000000000, 0.000000000000000000 ) ) ;
#20307=DIRECTION ( 'NONE',  ( 0.000000000000000000, 0.000000000000000000, -1.000000000000000000 ) ) ;
#20320=EDGE_LOOP ( 'NONE', ( #15944, #21002, #27600, #14068 ) ) ;
#20334=CARTESIAN_POINT ( 'NONE',  ( -0.3458446900868161200, 0.000000000000000000, -0.2204724409448818867 ) ) ;
#20438=EDGE_CURVE ( 'NONE', #10946, #18812, #8068, .T. ) ;
#20452=APPLICATION_CONTEXT ( 'automotive_design' ) ;
#20463=ORIENTED_EDGE ( 'NONE', *, *, #16639, .T. ) ;
#20507=DIRECTION ( 'NONE',  ( 0.000000000000000000, 0.000000000000000000, -1.000000000000000000 ) ) ;
#20520=AXIS2_PLACEMENT_3D ( 'NONE', #3774, #12394, #4198 ) ;
#20536=ADVANCED_FACE ( 'NONE', ( #12294, #7928 ), #24865, .T. ) ;
#20562=CARTESIAN_POINT ( 'NONE',  ( 0.000000000000000000, 0.000000000000000000, -0.1464516454673935042 ) ) ;
#20604=EDGE_LOOP ( 'NONE', ( #13360, #26147, #20463, #12232 ) ) ;
#20654=DIRECTION ( 'NONE',  ( 0.000000000000000000, 0.000000000000000000, 1.000000000000000000 ) ) ;
#20717=CARTESIAN_POINT ( 'NONE',  ( 0.000000000000000000, 0.000000000000000000, -0.2618110236220472231 ) ) ;
#20773=ORIENTED_EDGE ( 'NONE', *, *, #14472, .T. ) ;
#20795=CARTESIAN_POINT ( 'NONE',  ( 0.000000000000000000, 0.000000000000000000, -0.04133858267716535029 ) ) ;
#20862=TOROIDAL_SURFACE ( 'NONE', #14117, 0.3722026523000413478, 0.02755905511811023584 ) ;
#20884=EDGE_CURVE ( 'NONE', #25216, #3117, #25925, .T. ) ;
#20897=CIRCLE ( 'NONE', #8714, 0.4980314960629921295 ) ;
#20940=ADVANCED_FACE ( 'NONE', ( #17841 ), #13460, .T. ) ;
#20956=AXIS2_PLACEMENT_3D ( 'NONE', #21033, #19191, #21321 ) ;
#20957=CARTESIAN_POINT ( 'NONE',  ( 0.000000000000000000, 0.000000000000000000, -0.1464516454673935042 ) ) ;
#20969=EDGE_LOOP ( 'NONE', ( #2931, #7895, #19282, #22635 ) ) ;
#20993=EDGE_CURVE ( 'NONE', #19062, #19453, #4900, .T. ) ;
#21002=ORIENTED_EDGE ( 'NONE', *, *, #15459, .T. ) ;
#21009=CARTESIAN_POINT ( 'NONE',  ( 0.000000000000000000, 0.000000000000000000, -0.1559029880880275776 ) ) ;
#21033=CARTESIAN_POINT ( 'NONE',  ( -0.3866383478380992500, 0.000000000000000000, -0.2204724409448818867 ) ) ;
#21060=DIRECTION ( 'NONE',  ( 0.000000000000000000, 0.000000000000000000, -1.000000000000000000 ) ) ;
#21071=CARTESIAN_POINT ( 'NONE',  ( 2.185478346456692557E-17, -4.034314960629921845E-17, -0.1625845656552793450 ) ) ;
#21082=ORIENTED_EDGE ( 'NONE', *, *, #17516, .T. ) ;
#21086=DIRECTION ( 'NONE',  ( 1.000000000000000000, 0.000000000000000000, 0.000000000000000000 ) ) ;
#21094=ADVANCED_FACE ( 'NONE', ( #24346 ), #24762, .T. ) ;
#21195=PLANE ( 'NONE',  #18572 ) ;
#21200=CARTESIAN_POINT ( 'NONE',  ( -0.4685039370078740717, 0.000000000000000000, -0.01377952755905511792 ) ) ;
#21203=CONICAL_SURFACE ( 'NONE', #17583, 0.3039508883504944969, 0.2407725888118948110 ) ;
#21207=CARTESIAN_POINT ( 'NONE',  ( -0.3593781546376668135, 0.000000000000000000, -0.2755905511811023723 ) ) ;
#21250=ADVANCED_FACE ( 'NONE', ( #6961, #23652 ), #4818, .T. ) ;
#21321=DIRECTION ( 'NONE',  ( 1.000000000000000000, 0.000000000000000000, 0.000000000000000000 ) ) ;
#21326=AXIS2_PLACEMENT_3D ( 'NONE', #19917, #15956, #3078 ) ;
#21327=CARTESIAN_POINT ( 'NONE',  ( 0.000000000000000000, 0.000000000000000000, -0.1725236688546921415 ) ) ;
#21336=CARTESIAN_POINT ( 'NONE',  ( 0.000000000000000000, 0.000000000000000000, -0.2342519685039370358 ) ) ;
#21350=LINE ( 'NONE', #443, #6408 ) ;
#21413=DIRECTION ( 'NONE',  ( -1.000000000000000000, 0.000000000000000000, 0.000000000000000000 ) ) ;
#21421=AXIS2_PLACEMENT_3D ( 'NONE', #6772, #303, #26116 ) ;
#21442=EDGE_LOOP ( 'NONE', ( #6071, #2097 ) ) ;
#21499=DIRECTION ( 'NONE',  ( 0.000000000000000000, 0.000000000000000000, -1.000000000000000000 ) ) ;
#21501=DIRECTION ( 'NONE',  ( -1.000000000000000000, 0.000000000000000000, 0.000000000000000000 ) ) ;
#21521=DIRECTION ( 'NONE',  ( 1.000000000000000000, 0.000000000000000000, 0.000000000000000000 ) ) ;
#21537=( CONVERSION_BASED_UNIT ( 'INCH', #4306 ) LENGTH_UNIT ( ) NAMED_UNIT ( #12296 ) ) ;
#21554=CARTESIAN_POINT ( 'NONE',  ( 0.000000000000000000, -4.081314960629921056E-17, -0.1692378991623492424 ) ) ;
#21562=EDGE_CURVE ( 'NONE', #5769, #24896, #9080, .T. ) ;
#21568=EDGE_CURVE ( 'NONE', #26519, #17531, #21350, .T. ) ;
#21583=VECTOR ( 'NONE', #5792, 39.37007874015748854 ) ;
#21592=ORIENTED_EDGE ( 'NONE', *, *, #15719, .T. ) ;
#21615=CARTESIAN_POINT ( 'NONE',  ( -0.4010740433761567081, 0.000000000000000000, -0.2342519685039370358 ) ) ;
#21662=CARTESIAN_POINT ( 'NONE',  ( -0.3039508883504944969, 0.000000000000000000, -0.1111195235210984261 ) ) ;
#21702=DIRECTION ( 'NONE',  ( 0.000000000000000000, 0.000000000000000000, -1.000000000000000000 ) ) ;
#21806=CARTESIAN_POINT ( 'NONE',  ( 0.000000000000000000, 0.000000000000000000, -0.2342519685039370358 ) ) ;
#21813=( NAMED_UNIT ( * ) SI_UNIT ( $, .STERADIAN. ) SOLID_ANGLE_UNIT ( ) ) ;
#21881=CARTESIAN_POINT ( 'NONE',  ( 0.000000000000000000, 0.000000000000000000, -0.01377952755905511792 ) ) ;
#21905=DIRECTION ( 'NONE',  ( 0.000000000000000000, 0.000000000000000000, -1.000000000000000000 ) ) ;
#21913=EDGE_CURVE ( 'NONE', #8592, #1325, #7269, .T. ) ;
#22041=AXIS2_PLACEMENT_3D ( 'NONE', #19120, #27469, #17149 ) ;
#22058=ADVANCED_FACE ( 'NONE', ( #1759 ), #4391, .T. ) ;
#22111=AXIS2_PLACEMENT_3D ( 'NONE', #20957, #25188, #1459 ) ;
#22141=MANIFOLD_SOLID_BREP ( 'Shaft Seal 15x26x7', #18170 ) ;
#22160=CYLINDRICAL_SURFACE ( 'NONE', #11572, 0.3722026523000413478 ) ;
#22179=DIRECTION ( 'NONE',  ( 0.000000000000000000, 0.000000000000000000, -1.000000000000000000 ) ) ;
#22220=DIRECTION ( 'NONE',  ( 0.000000000000000000, 0.000000000000000000, -1.000000000000000000 ) ) ;
#22241=FACE_OUTER_BOUND ( 'NONE', #10412, .T. ) ;
#22257=CARTESIAN_POINT ( 'NONE',  ( 0.4980314960629921295, 6.183502046875907854E-17, -0.2755905511811023723 ) ) ;
#22260=AXIS2_PLACEMENT_3D ( 'NONE', #6882, #17735, #15383 ) ;
#22307=CARTESIAN_POINT ( 'NONE',  ( -0.4355945891378961154, 0.000000000000000000, -0.2755905511811023723 ) ) ;
#22322=VECTOR ( 'NONE', #16274, 39.37007874015748143 ) ;
#22371=VERTEX_POINT ( 'NONE', #21615 ) ;
#22396=DIRECTION ( 'NONE',  ( -1.000000000000000000, 0.000000000000000000, 0.000000000000000000 ) ) ;
#22401=ORIENTED_EDGE ( 'NONE', *, *, #19334, .F. ) ;
#22419=DIRECTION ( 'NONE',  ( -1.000000000000000000, -1.224646799147353454E-16, 0.000000000000000000 ) ) ;
#22519=EDGE_LOOP ( 'NONE', ( #12015, #24800, #6810, #7389 ) ) ;
#22528=AXIS2_PLACEMENT_3D ( 'NONE', #23139, #3619, #10259 ) ;
#22613=ORIENTED_EDGE ( 'NONE', *, *, #1096, .T. ) ;
#22635=ORIENTED_EDGE ( 'NONE', *, *, #3500, .F. ) ;
#22637=ADVANCED_FACE ( 'NONE', ( #7319 ), #7828, .F. ) ;
#22688=ORIENTED_EDGE ( 'NONE', *, *, #24229, .F. ) ;
#22704=AXIS2_PLACEMENT_3D ( 'NONE', #3632, #12258, #3928 ) ;
#22720=EDGE_LOOP ( 'NONE', ( #1664, #12952 ) ) ;
#22721=ORIENTED_EDGE ( 'NONE', *, *, #14932, .F. ) ;
#22805=EDGE_CURVE ( 'NONE', #1952, #18288, #19094, .T. ) ;
#22886=VECTOR ( 'NONE', #10450, 39.37007874015748854 ) ;
#22887=CARTESIAN_POINT ( 'NONE',  ( 0.000000000000000000, 0.000000000000000000, -0.1033464566929133965 ) ) ;
#22902=STYLED_ITEM ( 'NONE', ( #487 ), #22141 ) ;
#22938=ORIENTED_EDGE ( 'NONE', *, *, #5142, .F. ) ;
#22958=AXIS2_PLACEMENT_3D ( 'NONE', #21806, #19819, #19693 ) ;
#22966=EDGE_CURVE ( 'NONE', #17531, #10626, #8275, .T. ) ;
#23083=AXIS2_PLACEMENT_3D ( 'NONE', #20562, #26766, #22396 ) ;
#23087=LINE ( 'NONE', #25333, #9927 ) ;
#23139=CARTESIAN_POINT ( 'NONE',  ( 0.000000000000000000, 0.000000000000000000, -6.010066929133858501E-17 ) ) ;
#23164=CARTESIAN_POINT ( 'NONE',  ( 0.000000000000000000, -4.081314960629921056E-17, -0.1692378991623492424 ) ) ;
#23165=LINE ( 'NONE', #11998, #21583 ) ;
#23179=CARTESIAN_POINT ( 'NONE',  ( 0.000000000000000000, 0.000000000000000000, -0.01377952755905511792 ) ) ;
#23186=EDGE_LOOP ( 'NONE', ( #7429, #19284, #17638, #17470 ) ) ;
#23190=DIRECTION ( 'NONE',  ( 0.000000000000000000, 0.000000000000000000, -1.000000000000000000 ) ) ;
#23191=DIRECTION ( 'NONE',  ( 1.000000000000000000, 0.000000000000000000, 0.000000000000000000 ) ) ;
#23194=ORIENTED_EDGE ( 'NONE', *, *, #24462, .F. ) ;
#23222=CARTESIAN_POINT ( 'NONE',  ( 2.185478346456692557E-17, -4.034314960629921845E-17, -0.1625845656552793450 ) ) ;
#23223=DIRECTION ( 'NONE',  ( -1.000000000000000000, 0.000000000000000000, 0.000000000000000000 ) ) ;
#23372=FACE_BOUND ( 'NONE', #17893, .T. ) ;
#23377=CIRCLE ( 'NONE', #11167, 0.01377952755905510404 ) ;
#23390=CIRCLE ( 'NONE', #5841, 0.5118110236220472231 ) ;
#23459=PLANE ( 'NONE',  #20956 ) ;
#23470=FACE_OUTER_BOUND ( 'NONE', #6643, .T. ) ;
#23478=ORIENTED_EDGE ( 'NONE', *, *, #19902, .F. ) ;
#23487=CARTESIAN_POINT ( 'NONE',  ( -0.4980314960629921295, 0.000000000000000000, -0.2618110236220472231 ) ) ;
#23496=DIRECTION ( 'NONE',  ( 0.000000000000000000, 0.000000000000000000, -1.000000000000000000 ) ) ;
#23570=EDGE_CURVE ( 'NONE', #24185, #14002, #24061, .T. ) ;
#23574=ORIENTED_EDGE ( 'NONE', *, *, #4185, .T. ) ;
#23583=ORIENTED_EDGE ( 'NONE', *, *, #22966, .T. ) ;
#23622=DIRECTION ( 'NONE',  ( 0.5518027697606309179, -6.757634957480006187E-17, 0.8339746418713797071 ) ) ;
#23647=ADVANCED_FACE ( 'NONE', ( #1270 ), #25886, .T. ) ;
#23652=FACE_OUTER_BOUND ( 'NONE', #795, .T. ) ;
#23688=CIRCLE ( 'NONE', #10573, 0.3722026523000413478 ) ;
#23754=AXIS2_PLACEMENT_3D ( 'NONE', #13426, #26555, #11315 ) ;
#23773=PRODUCT_DEFINITION_FORMATION_WITH_SPECIFIED_SOURCE ( 'ANY', '', #3449, .NOT_KNOWN. ) ;
#23779=ADVANCED_FACE ( 'NONE', ( #17626 ), #10527, .F. ) ;
#23791=VERTEX_POINT ( 'NONE', #19472 ) ;
#23802=FILL_AREA_STYLE ('',( #19274 ) ) ;
#23833=EDGE_CURVE ( 'NONE', #23791, #10626, #26503, .T. ) ;
#23835=ORIENTED_EDGE ( 'NONE', *, *, #13862, .T. ) ;
#23873=CIRCLE ( 'NONE', #855, 0.3593781546537452298 ) ;
#23957=DIRECTION ( 'NONE',  ( -1.000000000000000000, 0.000000000000000000, 0.000000000000000000 ) ) ;
#24002=( LENGTH_UNIT ( ) NAMED_UNIT ( * ) SI_UNIT ( $, .METRE. ) ) ;
#24011=VERTEX_POINT ( 'NONE', #7075 ) ;
#24029=LINE ( 'NONE', #9047, #13702 ) ;
#24061=CIRCLE ( 'NONE', #18638, 0.3722026523000413478 ) ;
#24077=EDGE_LOOP ( 'NONE', ( #10692, #10108 ) ) ;
#24089=CARTESIAN_POINT ( 'NONE',  ( 0.000000000000000000, 0.000000000000000000, -0.1309055118110236116 ) ) ;
#24178=FACE_OUTER_BOUND ( 'NONE', #19073, .T. ) ;
#24185=VERTEX_POINT ( 'NONE', #16515 ) ;
#24205=CARTESIAN_POINT ( 'NONE',  ( 0.5118110236220472231, 6.267877318470705905E-17, -0.1377952755905511861 ) ) ;
#24208=DIRECTION ( 'NONE',  ( -1.000000000000000000, 0.000000000000000000, 0.000000000000000000 ) ) ;
#24229=EDGE_CURVE ( 'NONE', #24517, #22371, #15089, .T. ) ;
#24288=FACE_OUTER_BOUND ( 'NONE', #13532, .T. ) ;
#24292=VECTOR ( 'NONE', #10920, 39.37007874015748854 ) ;
#24302=LINE ( 'NONE', #17398, #1999 ) ;
#24325=AXIS2_PLACEMENT_3D ( 'NONE', #24089, #21702, #19851 ) ;
#24346=FACE_OUTER_BOUND ( 'NONE', #12498, .T. ) ;
#24398=DIRECTION ( 'NONE',  ( 0.000000000000000000, 0.000000000000000000, -1.000000000000000000 ) ) ;
#24420=FACE_OUTER_BOUND ( 'NONE', #1242, .T. ) ;
#24433=DIRECTION ( 'NONE',  ( 0.7212949172625979788, 8.833315116668955568E-17, -0.6926280692631088254 ) ) ;
#24447=ORIENTED_EDGE ( 'NONE', *, *, #5950, .T. ) ;
#24462=EDGE_CURVE ( 'NONE', #3117, #4205, #19136, .T. ) ;
#24473=ORIENTED_EDGE ( 'NONE', *, *, #24868, .F. ) ;
#24485=AXIS2_PLACEMENT_3D ( 'NONE', #6944, #4797, #15566 ) ;
#24489=ORIENTED_EDGE ( 'NONE', *, *, #15884, .T. ) ;
#24517=VERTEX_POINT ( 'NONE', #18667 ) ;
#24526=AXIS2_PLACEMENT_3D ( 'NONE', #20233, #749, #9338 ) ;
#24532=CARTESIAN_POINT ( 'NONE',  ( 0.000000000000000000, 0.000000000000000000, -0.2480314960629921295 ) ) ;
#24536=AXIS2_PLACEMENT_3D ( 'NONE', #21881, #24398, #13255 ) ;
#24588=AXIS2_PLACEMENT_3D ( 'NONE', #12197, #6516, #15146 ) ;
#24622=VERTEX_POINT ( 'NONE', #9770 ) ;
#24675=DIRECTION ( 'NONE',  ( 0.000000000000000000, 0.000000000000000000, -1.000000000000000000 ) ) ;
#24685=VERTEX_POINT ( 'NONE', #24696 ) ;
#24696=CARTESIAN_POINT ( 'NONE',  ( -0.4980314960629921295, 0.000000000000000000, -0.2755905511811023723 ) ) ;
#24733=DIRECTION ( 'NONE',  ( 0.000000000000000000, 0.000000000000000000, -1.000000000000000000 ) ) ;
#24739=ADVANCED_FACE ( 'NONE', ( #4362, #8187 ), #23459, .T. ) ;
#24762=CYLINDRICAL_SURFACE ( 'NONE', #14356, 0.5118110236220472231 ) ;
#24769=CARTESIAN_POINT ( 'NONE',  ( 0.3872945158171015589, 4.742989891227373650E-17, -0.2342519685039370358 ) ) ;
#24800=ORIENTED_EDGE ( 'NONE', *, *, #3260, .T. ) ;
#24808=FACE_OUTER_BOUND ( 'NONE', #18466, .T. ) ;
#24827=VERTEX_POINT ( 'NONE', #8053 ) ;
#24860=DIRECTION ( 'NONE',  ( 0.000000000000000000, 0.000000000000000000, -1.000000000000000000 ) ) ;
#24865=PLANE ( 'NONE',  #11651 ) ;
#24868=EDGE_CURVE ( 'NONE', #26728, #13078, #1556, .T. ) ;
#24871=ADVANCED_FACE ( 'NONE', ( #5038 ), #11468, .T. ) ;
#24894=CARTESIAN_POINT ( 'NONE',  ( -0.4763779527559054983, 0.000000000000000000, -0.01377952755905511792 ) ) ;
#24896=VERTEX_POINT ( 'NONE', #11267 ) ;
#24909=ORIENTED_EDGE ( 'NONE', *, *, #7871, .T. ) ;
#24991=EDGE_CURVE ( 'NONE', #27369, #7273, #25000, .T. ) ;
#24997=CIRCLE ( 'NONE', #24526, 0.4685039370078740717 ) ;
#25000=CIRCLE ( 'NONE', #645, 0.02755905511811020808 ) ;
#25004=FACE_OUTER_BOUND ( 'NONE', #27643, .T. ) ;
#25007=DIRECTION ( 'NONE',  ( -1.000000000000000000, -1.224646799147356165E-16, 0.000000000000000000 ) ) ;
#25044=DIRECTION ( 'NONE',  ( 0.000000000000000000, 0.000000000000000000, 1.000000000000000000 ) ) ;
#25084=DIRECTION ( 'NONE',  ( 0.000000000000000000, 0.000000000000000000, -1.000000000000000000 ) ) ;
#25087=DIRECTION ( 'NONE',  ( 0.000000000000000000, 0.000000000000000000, -1.000000000000000000 ) ) ;
#25142=ORIENTED_EDGE ( 'NONE', *, *, #24991, .F. ) ;
#25171=CIRCLE ( 'NONE', #12548, 0.01377952755905510404 ) ;
#25173=CIRCLE ( 'NONE', #27006, 0.2952755905511810774 ) ;
#25188=DIRECTION ( 'NONE',  ( 0.000000000000000000, 0.000000000000000000, -1.000000000000000000 ) ) ;
#25216=VERTEX_POINT ( 'NONE', #10247 ) ;
#25276=CARTESIAN_POINT ( 'NONE',  ( 0.000000000000000000, 0.000000000000000000, -0.05511811023622047168 ) ) ;
#25284=DIRECTION ( 'NONE',  ( -1.000000000000000000, 0.000000000000000000, 0.000000000000000000 ) ) ;
#25333=CARTESIAN_POINT ( 'NONE',  ( 0.3039508883504944969, 3.722324825164276661E-17, -0.1111195235210984261 ) ) ;
#25383=EDGE_CURVE ( 'NONE', #3782, #13078, #15569, .T. ) ;
#25436=CARTESIAN_POINT ( 'NONE',  ( 0.5118110236220472231, 6.267877318470705905E-17, -0.01377952755905511792 ) ) ;
#25493=EDGE_CURVE ( 'NONE', #22371, #10946, #14301, .T. ) ;
#25527=FACE_OUTER_BOUND ( 'NONE', #22519, .T. ) ;
#25560=DIRECTION ( 'NONE',  ( -0.000000000000000000, -1.000000000000000000, -0.000000000000000000 ) ) ;
#25585=EDGE_CURVE ( 'NONE', #14002, #9997, #3246, .T. ) ;
#25589=DIRECTION ( 'NONE',  ( 1.000000000000000000, 0.000000000000000000, 0.000000000000000000 ) ) ;
#25630=CIRCLE ( 'NONE', #11619, 0.02755905511811023931 ) ;
#25686=ORIENTED_EDGE ( 'NONE', *, *, #24868, .T. ) ;
#25705=DIRECTION ( 'NONE',  ( 0.000000000000000000, 0.000000000000000000, -1.000000000000000000 ) ) ;
#25717=CARTESIAN_POINT ( 'NONE',  ( -0.3224687058348476576, 0.000000000000000000, -0.1559029880880275776 ) ) ;
#25731=ORIENTED_EDGE ( 'NONE', *, *, #15884, .F. ) ;
#25798=SHAPE_REPRESENTATION ( 'Shaft Seal 15x26x7', ( #11588 ), #6215 ) ;
#25877=DIRECTION ( 'NONE',  ( -1.000000000000000000, 0.000000000000000000, 0.000000000000000000 ) ) ;
#25886=TOROIDAL_SURFACE ( 'NONE', #12345, 0.3722026523000413478, 0.02755905511811023584 ) ;
#25907=CARTESIAN_POINT ( 'NONE',  ( 0.000000000000000000, 0.000000000000000000, -0.1559029880880275776 ) ) ;
#25925=LINE ( 'NONE', #26459, #4011 ) ;
#25982=DIRECTION ( 'NONE',  ( 0.000000000000000000, 0.000000000000000000, -1.000000000000000000 ) ) ;
#25992=FACE_OUTER_BOUND ( 'NONE', #14887, .T. ) ;
#26038=AXIS2_PLACEMENT_3D ( 'NONE', #6511, #15143, #12996 ) ;
#26084=EDGE_CURVE ( 'NONE', #24622, #20206, #3364, .T. ) ;
#26116=DIRECTION ( 'NONE',  ( 1.000000000000000000, 0.000000000000000000, 0.000000000000000000 ) ) ;
#26147=ORIENTED_EDGE ( 'NONE', *, *, #4258, .T. ) ;
#26148=FACE_OUTER_BOUND ( 'NONE', #9870, .T. ) ;
#26158=ADVANCED_FACE ( 'NONE', ( #24288 ), #26271, .T. ) ;
#26182=ADVANCED_BREP_SHAPE_REPRESENTATION ( 'Shaft Seal 15x26x7', ( #22141, #11588 ), #6215 ) ;
#26187=FACE_OUTER_BOUND ( 'NONE', #1534, .T. ) ;
#26193=ORIENTED_EDGE ( 'NONE', *, *, #862, .T. ) ;
#26202=DIRECTION ( 'NONE',  ( 0.000000000000000000, 0.000000000000000000, -1.000000000000000000 ) ) ;
#26267=DIRECTION ( 'NONE',  ( 1.000000000000000000, 0.000000000000000000, 0.000000000000000000 ) ) ;
#26271=CYLINDRICAL_SURFACE ( 'NONE', #15169, 0.3722026523000413478 ) ;
#26299=LINE ( 'NONE', #21662, #24292 ) ;
#26377=CARTESIAN_POINT ( 'NONE',  ( 0.000000000000000000, 0.000000000000000000, -0.1725236688546921415 ) ) ;
#26391=CARTESIAN_POINT ( 'NONE',  ( 0.000000000000000000, 0.000000000000000000, -0.05856299212598425896 ) ) ;
#26442=DIRECTION ( 'NONE',  ( 1.000000000000000000, 0.000000000000000000, 0.000000000000000000 ) ) ;
#26444=ORIENTED_EDGE ( 'NONE', *, *, #5142, .T. ) ;
#26459=CARTESIAN_POINT ( 'NONE',  ( -0.3722026523000413478, 0.000000000000000000, -0.1756889763779527769 ) ) ;
#26461=CIRCLE ( 'NONE', #26038, 0.3593781546537452298 ) ;
#26468=LINE ( 'NONE', #26898, #14330 ) ;
#26503=LINE ( 'NONE', #1103, #9603 ) ;
#26519=VERTEX_POINT ( 'NONE', #11590 ) ;
#26554=AXIS2_PLACEMENT_3D ( 'NONE', #17816, #4971, #359 ) ;
#26555=DIRECTION ( 'NONE',  ( 0.000000000000000000, 0.000000000000000000, -1.000000000000000000 ) ) ;
#26595=CIRCLE ( 'NONE', #10355, 0.01377952755905511792 ) ;
#26597=ADVANCED_FACE ( 'NONE', ( #24178 ), #4813, .F. ) ;
#26653=DIRECTION ( 'NONE',  ( -1.000000000000000000, 0.000000000000000000, 0.000000000000000000 ) ) ;
#26659=ORIENTED_EDGE ( 'NONE', *, *, #4744, .T. ) ;
#26660=ADVANCED_FACE ( 'NONE', ( #25004 ), #5668, .T. ) ;
#26661=DIRECTION ( 'NONE',  ( -1.000000000000000000, 0.000000000000000000, 0.000000000000000000 ) ) ;
#26708=CARTESIAN_POINT ( 'NONE',  ( -0.3722026523000413478, 0.000000000000000000, -0.07578740157480315376 ) ) ;
#26728=VERTEX_POINT ( 'NONE', #5526 ) ;
#26766=DIRECTION ( 'NONE',  ( 0.000000000000000000, 0.000000000000000000, -1.000000000000000000 ) ) ;
#26767=ORIENTED_EDGE ( 'NONE', *, *, #17887, .F. ) ;
#26821=DIRECTION ( 'NONE',  ( 0.000000000000000000, 0.000000000000000000, 1.000000000000000000 ) ) ;
#26895=ORIENTED_EDGE ( 'NONE', *, *, #3260, .F. ) ;
#26898=CARTESIAN_POINT ( 'NONE',  ( 0.4842519685039370358, 5.930376232091513698E-17, -0.1309055118110236116 ) ) ;
#26899=DIRECTION ( 'NONE',  ( 0.000000000000000000, 0.000000000000000000, -1.000000000000000000 ) ) ;
#26903=AXIS2_PLACEMENT_3D ( 'NONE', #23222, #12472, #21086 ) ;
#26909=VERTEX_POINT ( 'NONE', #25436 ) ;
#26917=AXIS2_PLACEMENT_3D ( 'NONE', #24769, #5435, #16025 ) ;
#26939=CARTESIAN_POINT ( 'NONE',  ( -0.3722026523000413478, 0.000000000000000000, -0.2204724409448818867 ) ) ;
#27006=AXIS2_PLACEMENT_3D ( 'NONE', #10755, #21499, #6522 ) ;
#27105=DIRECTION ( 'NONE',  ( 0.000000000000000000, 0.000000000000000000, -1.000000000000000000 ) ) ;
#27128=DIRECTION ( 'NONE',  ( 1.000000000000000000, 0.000000000000000000, 0.000000000000000000 ) ) ;
#27170=DIRECTION ( 'NONE',  ( 1.000000000000000000, 0.000000000000000000, 0.000000000000000000 ) ) ;
#27208=CARTESIAN_POINT ( 'NONE',  ( -0.3584231247409862542, 0.000000000000000000, -0.04133858267716535029 ) ) ;
#27226=CARTESIAN_POINT ( 'NONE',  ( 0.3332647802741406373, 4.241214765863767561E-17, -0.1692378991623492424 ) ) ;
#27259=CIRCLE ( 'NONE', #10555, 0.3722026523000413478 ) ;
#27265=ADVANCED_FACE ( 'NONE', ( #17038 ), #18716, .F. ) ;
#27280=VECTOR ( 'NONE', #821, 39.37007874015748143 ) ;
#27332=ADVANCED_FACE ( 'NONE', ( #2320 ), #376, .F. ) ;
#27369=VERTEX_POINT ( 'NONE', #254 ) ;
#27407=DIRECTION ( 'NONE',  ( 0.000000000000000000, 0.000000000000000000, -1.000000000000000000 ) ) ;
#27421=CYLINDRICAL_SURFACE ( 'NONE', #9982, 0.3722026523000413478 ) ;
#27450=DIRECTION ( 'NONE',  ( 1.000000000000000000, 0.000000000000000000, 0.000000000000000000 ) ) ;
#27469=DIRECTION ( 'NONE',  ( 0.000000000000000000, 0.000000000000000000, -1.000000000000000000 ) ) ;
#27600=ORIENTED_EDGE ( 'NONE', *, *, #23833, .T. ) ;
#27643=EDGE_LOOP ( 'NONE', ( #4034, #24489, #7294, #1887 ) ) ;
#27654=ORIENTED_EDGE ( 'NONE', *, *, #24462, .T. ) ;
#27664=ORIENTED_EDGE ( 'NONE', *, *, #5950, .F. ) ;
#27677=DIRECTION ( 'NONE',  ( 1.000000000000000000, 0.000000000000000000, 0.000000000000000000 ) ) ;
#27690=AXIS2_PLACEMENT_3D ( 'NONE', #2841, #2334, #11612 ) ;
#27696=CARTESIAN_POINT ( 'NONE',  ( 0.000000000000000000, 0.000000000000000000, -0.07578740157480315376 ) ) ;
#27699=EDGE_CURVE ( 'NONE', #16461, #12825, #26461, .T. ) ;
#27735=CIRCLE ( 'NONE', #24536, 0.4842519685039370358 ) ;
#27740=CARTESIAN_POINT ( 'NONE',  ( 0.000000000000000000, 0.000000000000000000, -0.2204724409448818867 ) ) ;
#27741=CARTESIAN_POINT ( 'NONE',  ( 0.000000000000000000, 0.000000000000000000, -0.2204724409448818867 ) ) ;
#27824=DIRECTION ( 'NONE',  ( 0.000000000000000000, 0.000000000000000000, -1.000000000000000000 ) ) ;
ENDSEC;
END-ISO-10303-21;
